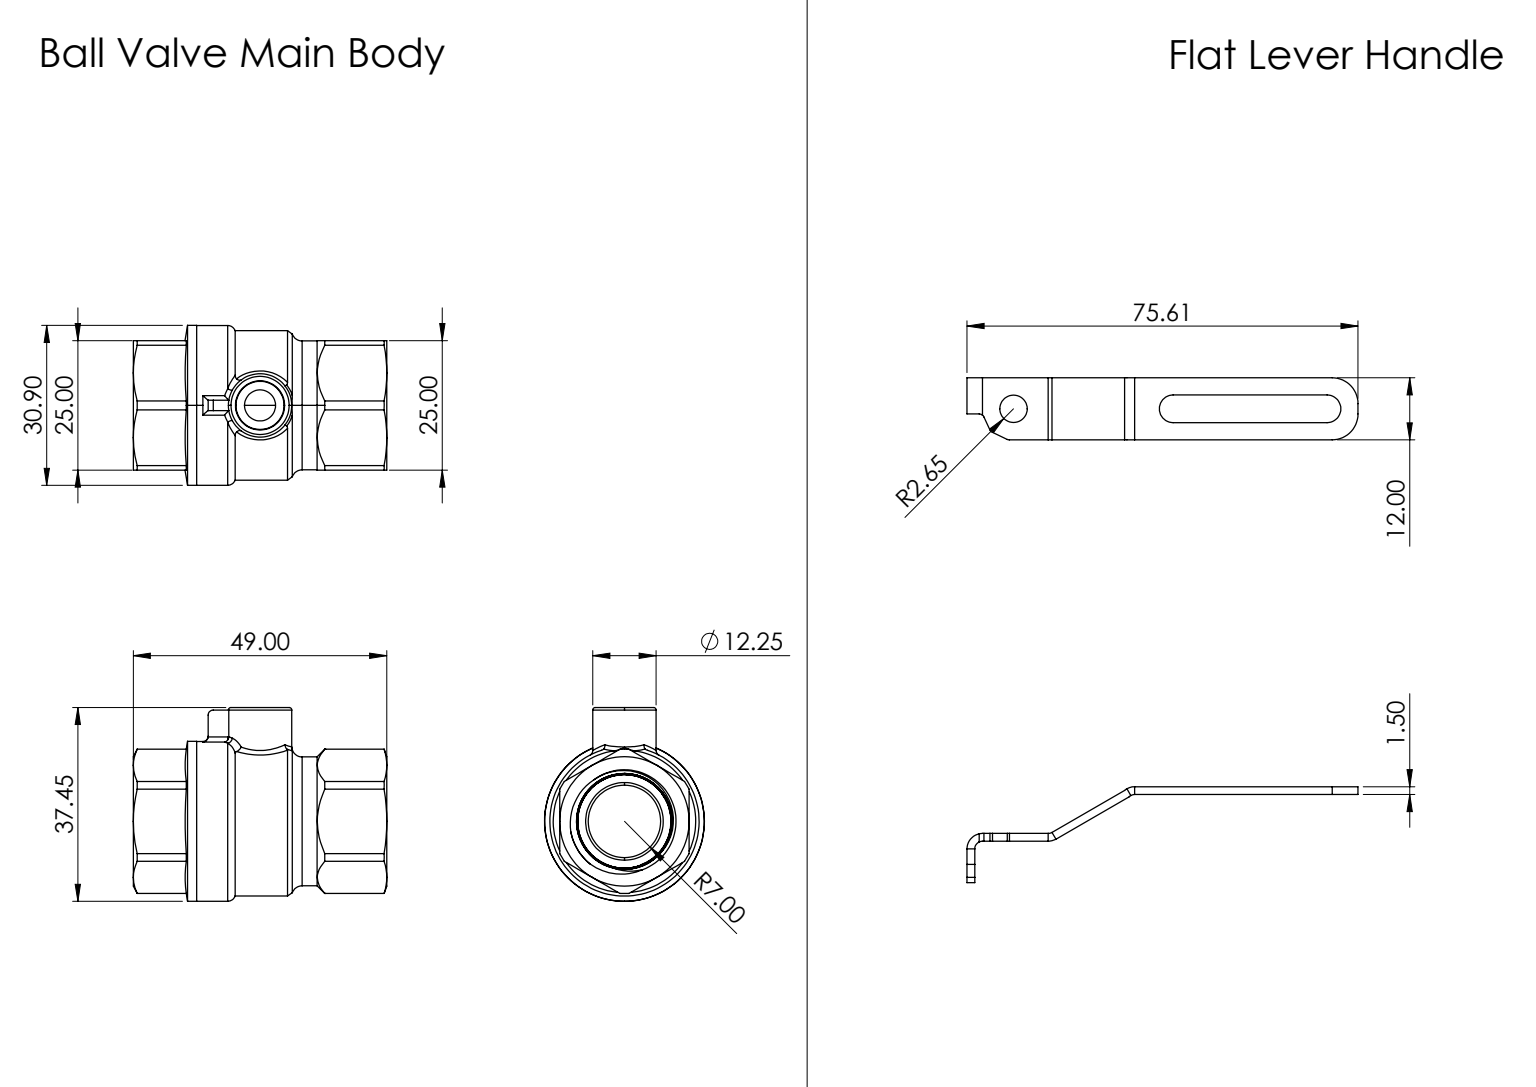
ISO-10303-21;
HEADER;
FILE_DESCRIPTION (('STEP AP214'),
    '1' );
FILE_NAME ('Flat Lever Handle.step',
    '2026-10-09T13:48:35',
    ( '' ),
    ( '' ),
    'SwSTEP 2.0',
    'SolidWorks 2026',
    '' );
FILE_SCHEMA (( 'AUTOMOTIVE_DESIGN' ));
ENDSEC;

DATA;
#4=DIRECTION ( 'NONE',  ( 1.000000000000000000, 0.000000000000000000, 0.000000000000000000 ) ) ;
#6=EDGE_LOOP ( 'NONE', ( #5081, #3644, #13220, #12725 ) ) ;
#25=AXIS2_PLACEMENT_3D ( 'NONE', #17058, #6275, #4594 ) ;
#141=CARTESIAN_POINT ( 'NONE',  ( -130.2348000000000070, 19.50000000000000000, -2.000000000000000000 ) ) ;
#152=CIRCLE ( 'NONE', #7126, 1.500000000000001332 ) ;
#154=EDGE_CURVE ( 'NONE', #7280, #18990, #3410, .T. ) ;
#165=VERTEX_POINT ( 'NONE', #14005 ) ;
#197=DIRECTION ( 'NONE',  ( 0.000000000000000000, 1.000000000000000000, 0.000000000000000000 ) ) ;
#205=ORIENTED_EDGE ( 'NONE', *, *, #8949, .F. ) ;
#208=EDGE_CURVE ( 'NONE', #14474, #22330, #6328, .T. ) ;
#229=DIRECTION ( 'NONE',  ( -0.5000000000000169864, 0.8660254037844288266, 0.000000000000000000 ) ) ;
#230=ORIENTED_EDGE ( 'NONE', *, *, #502, .T. ) ;
#262=LINE ( 'NONE', #11311, #3334 ) ;
#289=DIRECTION ( 'NONE',  ( 1.000000000000000000, 0.000000000000000000, 0.000000000000000000 ) ) ;
#311=VECTOR ( 'NONE', #7009, 1000.000000000000000 ) ;
#329=FACE_OUTER_BOUND ( 'NONE', #10599, .T. ) ;
#332=CYLINDRICAL_SURFACE ( 'NONE', #6125, 2.649999999999999911 ) ;
#336=CLOSED_SHELL ( 'NONE', ( #19786, #22741, #8979, #14137, #5705, #10585, #19906, #17710, #15034, #14866, #16344, #2572, #1995, #20352, #20018, #16952, #22187, #19348, #3814, #13211, #2540, #15971, #923, #17120, #9106, #4929, #6763, #19413, #8384, #21247, #11430, #1672, #12020, #13623, #15533, #9283, #9847, #3649, #4205, #7320, #9527, #23189, #20165, #21835, #18823, #16204, #1398 ) ) ;
#371=PLANE ( 'NONE',  #4207 ) ;
#399=ORIENTED_EDGE ( 'NONE', *, *, #17076, .T. ) ;
#408=CARTESIAN_POINT ( 'NONE',  ( -9.000000000000000000, 19.50000000000000000, -1.000000000000000000 ) ) ;
#412=AXIS2_PLACEMENT_3D ( 'NONE', #8961, #23955, #5663 ) ;
#424=CARTESIAN_POINT ( 'NONE',  ( 23.75352077758000036, 36.75000000000000000, 6.000000000000000000 ) ) ;
#427=CYLINDRICAL_SURFACE ( 'NONE', #12766, 2.999999999999999112 ) ;
#434=FACE_OUTER_BOUND ( 'NONE', #19147, .T. ) ;
#470=DIRECTION ( 'NONE',  ( 0.000000000000000000, 1.000000000000000000, 0.000000000000000000 ) ) ;
#483=PRODUCT ( 'Flat Lever Handle', 'Flat Lever Handle', '', ( #22105 ) ) ;
#502=EDGE_CURVE ( 'NONE', #22896, #18160, #1313, .T. ) ;
#506=CARTESIAN_POINT ( 'NONE',  ( -7.500000000000000000, 22.00000000000000000, 1.000000000000000000 ) ) ;
#512=ORIENTED_EDGE ( 'NONE', *, *, #10459, .F. ) ;
#531=DIRECTION ( 'NONE',  ( 0.8660254037844288266, 0.5000000000000169864, 0.000000000000000000 ) ) ;
#535=CARTESIAN_POINT ( 'NONE',  ( -9.000000000000000000, 18.50000000000000000, -5.000000000000000000 ) ) ;
#537=EDGE_CURVE ( 'NONE', #23889, #15891, #18705, .T. ) ;
#545=ORIENTED_EDGE ( 'NONE', *, *, #18849, .F. ) ;
#560=DIRECTION ( 'NONE',  ( 0.000000000000000000, 0.000000000000000000, -1.000000000000000000 ) ) ;
#582=ORIENTED_EDGE ( 'NONE', *, *, #5142, .F. ) ;
#583=EDGE_CURVE ( 'NONE', #14220, #9013, #21124, .T. ) ;
#589=DIRECTION ( 'NONE',  ( -0.5000000000000169864, 0.8660254037844288266, 0.000000000000000000 ) ) ;
#611=VERTEX_POINT ( 'NONE', #13485 ) ;
#615=ORIENTED_EDGE ( 'NONE', *, *, #5201, .F. ) ;
#634=EDGE_CURVE ( 'NONE', #15280, #17036, #9741, .T. ) ;
#637=CARTESIAN_POINT ( 'NONE',  ( 23.41677564524290744, 35.51856778792605240, -6.000000000000000000 ) ) ;
#640=ORIENTED_EDGE ( 'NONE', *, *, #17076, .F. ) ;
#641=CYLINDRICAL_SURFACE ( 'NONE', #10623, 1.000000000000000888 ) ;
#653=CARTESIAN_POINT ( 'NONE',  ( 7.446152422707000618, 28.20096189432300093, 6.000000000000000000 ) ) ;
#677=ORIENTED_EDGE ( 'NONE', *, *, #17568, .T. ) ;
#722=PLANE ( 'NONE',  #6401 ) ;
#728=ORIENTED_EDGE ( 'NONE', *, *, #1649, .T. ) ;
#729=VECTOR ( 'NONE', #20922, 1000.000000000000000 ) ;
#732=DIRECTION ( 'NONE',  ( 0.000000000000000000, -1.000000000000000000, 1.361873576874000145E-14 ) ) ;
#734=AXIS2_PLACEMENT_3D ( 'NONE', #10520, #4708, #10636 ) ;
#736=DIRECTION ( 'NONE',  ( 0.8660254037844288266, 0.5000000000000169864, 0.000000000000000000 ) ) ;
#773=DIRECTION ( 'NONE',  ( 0.000000000000000000, -1.000000000000000000, 0.000000000000000000 ) ) ;
#789=FACE_OUTER_BOUND ( 'NONE', #3552, .T. ) ;
#793=FACE_OUTER_BOUND ( 'NONE', #14111, .T. ) ;
#808=EDGE_CURVE ( 'NONE', #11090, #23810, #13051, .T. ) ;
#823=ORIENTED_EDGE ( 'NONE', *, *, #5689, .F. ) ;
#860=CARTESIAN_POINT ( 'NONE',  ( -6.000000000000000000, 28.00000000000000000, 1.229194263906999929 ) ) ;
#864=CARTESIAN_POINT ( 'NONE',  ( 7.446152422707000618, 28.20096189432300093, -6.000000000000000000 ) ) ;
#881=LINE ( 'NONE', #11679, #5311 ) ;
#923=ADVANCED_FACE ( 'NONE', ( #1624 ), #23661, .F. ) ;
#932=VECTOR ( 'NONE', #12319, 1000.000000000000000 ) ;
#962=FACE_OUTER_BOUND ( 'NONE', #5721, .T. ) ;
#983=PLANE ( 'NONE',  #23592 ) ;
#1009=CIRCLE ( 'NONE', #16482, 5.000000000000000000 ) ;
#1013=CARTESIAN_POINT ( 'NONE',  ( 23.41677564524290744, 34.01856778792605240, 6.000000000000000000 ) ) ;
#1042=CARTESIAN_POINT ( 'NONE',  ( 60.61494135913342518, 27.01856778792605240, -2.673746900119611247 ) ) ;
#1047=AXIS2_PLACEMENT_3D ( 'NONE', #19546, #12406, #6941 ) ;
#1061=DIRECTION ( 'NONE',  ( 1.000000000000000000, 0.000000000000000000, -1.253337711393242021E-14 ) ) ;
#1093=DIRECTION ( 'NONE',  ( 1.000000000000000000, 0.000000000000000000, 0.000000000000000000 ) ) ;
#1107=VECTOR ( 'NONE', #14524, 1000.000000000000000 ) ;
#1126=ORIENTED_EDGE ( 'NONE', *, *, #3156, .T. ) ;
#1130=ORIENTED_EDGE ( 'NONE', *, *, #7876, .F. ) ;
#1136=CARTESIAN_POINT ( 'NONE',  ( -3.657438266360000245, 28.00000000000000000, 3.657438266360000245 ) ) ;
#1226=CARTESIAN_POINT ( 'NONE',  ( 30.87226923053214378, 37.01856778792605240, -2.673746900119611247 ) ) ;
#1243=CARTESIAN_POINT ( 'NONE',  ( -7.500000000000000000, 18.50000000000000000, -5.000000000000000000 ) ) ;
#1253=ORIENTED_EDGE ( 'NONE', *, *, #13521, .F. ) ;
#1276=EDGE_CURVE ( 'NONE', #9702, #13003, #19100, .T. ) ;
#1285=ORIENTED_EDGE ( 'NONE', *, *, #583, .F. ) ;
#1290=ORIENTED_EDGE ( 'NONE', *, *, #154, .F. ) ;
#1301=DIRECTION ( 'NONE',  ( 0.000000000000000000, 0.000000000000000000, -1.000000000000000000 ) ) ;
#1313=CIRCLE ( 'NONE', #11367, 0.9999999999999995559 ) ;
#1318=FACE_OUTER_BOUND ( 'NONE', #12289, .T. ) ;
#1332=AXIS2_PLACEMENT_3D ( 'NONE', #10810, #12736, #5236 ) ;
#1336=ORIENTED_EDGE ( 'NONE', *, *, #20077, .F. ) ;
#1348=EDGE_LOOP ( 'NONE', ( #23222, #2521, #7520, #9139 ) ) ;
#1352=FACE_OUTER_BOUND ( 'NONE', #11148, .T. ) ;
#1359=DIRECTION ( 'NONE',  ( 0.000000000000000000, 0.000000000000000000, 1.000000000000000000 ) ) ;
#1360=VERTEX_POINT ( 'NONE', #23263 ) ;
#1373=CARTESIAN_POINT ( 'NONE',  ( -9.000000000000000000, 19.50000000000000000, -1.000000000000000000 ) ) ;
#1398=ADVANCED_FACE ( 'NONE', ( #18306 ), #5347, .F. ) ;
#1449=ORIENTED_EDGE ( 'NONE', *, *, #13356, .F. ) ;
#1459=CARTESIAN_POINT ( 'NONE',  ( 23.41677564524290744, 37.01856778792605240, -6.000000000000000000 ) ) ;
#1470=ORIENTED_EDGE ( 'NONE', *, *, #634, .T. ) ;
#1529=AXIS2_PLACEMENT_3D ( 'NONE', #6973, #16287, #9266 ) ;
#1538=FACE_OUTER_BOUND ( 'NONE', #11239, .T. ) ;
#1541=EDGE_CURVE ( 'NONE', #13175, #5360, #5876, .T. ) ;
#1546=CARTESIAN_POINT ( 'NONE',  ( 2.649999999999999911, 28.00000000000000000, 0.000000000000000000 ) ) ;
#1571=CYLINDRICAL_SURFACE ( 'NONE', #15011, 2.673746900119611247 ) ;
#1576=CARTESIAN_POINT ( 'NONE',  ( 66.60588651278291650, 37.01856778792605240, 1.000000000000000000 ) ) ;
#1602=CARTESIAN_POINT ( 'NONE',  ( 60.61494135913342518, 27.01856778792605240, 2.673746900119611247 ) ) ;
#1616=ORIENTED_EDGE ( 'NONE', *, *, #7937, .F. ) ;
#1619=DIRECTION ( 'NONE',  ( 0.000000000000000000, 1.000000000000000000, 0.000000000000000000 ) ) ;
#1621=ORIENTED_EDGE ( 'NONE', *, *, #21569, .T. ) ;
#1624=FACE_OUTER_BOUND ( 'NONE', #21156, .T. ) ;
#1625=ORIENTED_EDGE ( 'NONE', *, *, #4322, .T. ) ;
#1639=ORIENTED_EDGE ( 'NONE', *, *, #2556, .F. ) ;
#1649=EDGE_CURVE ( 'NONE', #13003, #12335, #9333, .T. ) ;
#1667=EDGE_LOOP ( 'NONE', ( #1625, #4186, #23393, #4526 ) ) ;
#1671=EDGE_LOOP ( 'NONE', ( #5379, #9334, #2085, #16002 ) ) ;
#1672=ADVANCED_FACE ( 'NONE', ( #11276 ), #14887, .F. ) ;
#1674=CARTESIAN_POINT ( 'NONE',  ( -6.637070260807000466, 27.93157662065900126, 1.000000000000000000 ) ) ;
#1689=FACE_BOUND ( 'NONE', #22379, .T. ) ;
#1737=EDGE_CURVE ( 'NONE', #1360, #17036, #8351, .T. ) ;
#1739=CIRCLE ( 'NONE', #12188, 1.000000000000000888 ) ;
#1756=ORIENTED_EDGE ( 'NONE', *, *, #16140, .T. ) ;
#1764=VECTOR ( 'NONE', #4364, 1000.000000000000000 ) ;
#1771=EDGE_CURVE ( 'NONE', #6372, #15650, #8993, .T. ) ;
#1792=DIRECTION ( 'NONE',  ( 0.000000000000000000, 0.000000000000000000, 1.000000000000000000 ) ) ;
#1824=ORIENTED_EDGE ( 'NONE', *, *, #23121, .T. ) ;
#1840=PLANE ( 'NONE',  #16418 ) ;
#1847=CARTESIAN_POINT ( 'NONE',  ( -7.500000000000000000, 18.50000000000000000, -2.000000000000000000 ) ) ;
#1861=DIRECTION ( 'NONE',  ( 0.000000000000000000, -1.000000000000000000, 0.000000000000000000 ) ) ;
#1876=MECHANICAL_DESIGN_GEOMETRIC_PRESENTATION_REPRESENTATION('',(#8060),#12344);
#1896=DIRECTION ( 'NONE',  ( -0.000000000000000000, 1.000000000000000000, -0.000000000000000000 ) ) ;
#1905=VECTOR ( 'NONE', #20072, 1000.000000000000000 ) ;
#1971=ORIENTED_EDGE ( 'NONE', *, *, #154, .T. ) ;
#1977=EDGE_CURVE ( 'NONE', #5360, #13125, #15211, .T. ) ;
#1995=ADVANCED_FACE ( 'NONE', ( #2386 ), #3858, .F. ) ;
#1998=PRODUCT_DEFINITION_CONTEXT ( 'detailed design', #23802, 'design' ) ;
#2000=DIRECTION ( 'NONE',  ( 0.000000000000000000, -1.000000000000000000, 0.000000000000000000 ) ) ;
#2012=LINE ( 'NONE', #23616, #6899 ) ;
#2020=CARTESIAN_POINT ( 'NONE',  ( -3.657438266360000245, 26.50000000000000000, 3.657438266360000245 ) ) ;
#2038=DIRECTION ( 'NONE',  ( 0.000000000000000000, -1.000000000000000000, 0.000000000000000000 ) ) ;
#2085=ORIENTED_EDGE ( 'NONE', *, *, #10886, .T. ) ;
#2090=ORIENTED_EDGE ( 'NONE', *, *, #3850, .F. ) ;
#2136=CARTESIAN_POINT ( 'NONE',  ( -6.525832981339341643, 26.41017609473133732, 0.9999999999999872324 ) ) ;
#2157=PLANE ( 'NONE',  #9897 ) ;
#2190=CARTESIAN_POINT ( 'NONE',  ( 60.61494135913342518, 35.51856778792605240, 2.673746900119610359 ) ) ;
#2196=DIRECTION ( 'NONE',  ( 0.000000000000000000, 0.000000000000000000, -1.000000000000000000 ) ) ;
#2205=DIRECTION ( 'NONE',  ( 0.000000000000000000, -1.000000000000000000, 0.000000000000000000 ) ) ;
#2209=DIRECTION ( 'NONE',  ( 0.000000000000000000, 0.000000000000000000, 1.000000000000000000 ) ) ;
#2241=DIRECTION ( 'NONE',  ( 1.000000000000000000, 0.000000000000000000, 0.000000000000000000 ) ) ;
#2243=ORIENTED_EDGE ( 'NONE', *, *, #13378, .T. ) ;
#2262=CIRCLE ( 'NONE', #11164, 1.500000000000001332 ) ;
#2276=VECTOR ( 'NONE', #589, 1000.000000000000114 ) ;
#2284=ORIENTED_EDGE ( 'NONE', *, *, #20180, .T. ) ;
#2317=CARTESIAN_POINT ( 'NONE',  ( 23.01485185659291233, 37.01856778792605240, -6.000000000000000000 ) ) ;
#2318=ORIENTED_EDGE ( 'NONE', *, *, #537, .T. ) ;
#2350=DIRECTION ( 'NONE',  ( 0.000000000000000000, -1.000000000000000000, 0.000000000000000000 ) ) ;
#2356=DIRECTION ( 'NONE',  ( -1.387778780781444413E-14, 1.000000000000000000, 0.000000000000000000 ) ) ;
#2373=DIRECTION ( 'NONE',  ( 0.000000000000000000, 0.000000000000000000, -1.000000000000000000 ) ) ;
#2374=VERTEX_POINT ( 'NONE', #18954 ) ;
#2386=FACE_OUTER_BOUND ( 'NONE', #10840, .T. ) ;
#2399=CARTESIAN_POINT ( 'NONE',  ( -6.637070260807000466, 26.35799170939839797, 1.000000000000000000 ) ) ;
#2425=DIRECTION ( 'NONE',  ( 0.9063077870366409439, 0.000000000000000000, -0.4226182617407189257 ) ) ;
#2465=CARTESIAN_POINT ( 'NONE',  ( 8.196152422706999729, 26.90192378864669820, -6.000000000000000000 ) ) ;
#2473=AXIS2_PLACEMENT_3D ( 'NONE', #2819, #1359, #21464 ) ;
#2501=AXIS2_PLACEMENT_3D ( 'NONE', #7515, #2425, #9577 ) ;
#2521=ORIENTED_EDGE ( 'NONE', *, *, #18719, .F. ) ;
#2529=VECTOR ( 'NONE', #15495, 1000.000000000000000 ) ;
#2540=ADVANCED_FACE ( 'NONE', ( #23055 ), #15665, .T. ) ;
#2556=EDGE_CURVE ( 'NONE', #18990, #5263, #11534, .T. ) ;
#2572=ADVANCED_FACE ( 'NONE', ( #3789 ), #13104, .F. ) ;
#2591=CARTESIAN_POINT ( 'NONE',  ( -7.500000000000000000, 22.00000000000000000, 1.000000000000000000 ) ) ;
#2603=AXIS2_PLACEMENT_3D ( 'NONE', #5656, #9656, #20438 ) ;
#2616=LINE ( 'NONE', #8311, #4226 ) ;
#2620=CARTESIAN_POINT ( 'NONE',  ( -6.199443458293737663, 26.48693030808626503, 1.100246419409809828 ) ) ;
#2655=PLANE ( 'NONE',  #4969 ) ;
#2658=DIRECTION ( 'NONE',  ( 0.000000000000000000, 1.000000000000000000, 0.000000000000000000 ) ) ;
#2660=ORIENTED_EDGE ( 'NONE', *, *, #12790, .F. ) ;
#2681=VERTEX_POINT ( 'NONE', #13452 ) ;
#2688=CARTESIAN_POINT ( 'NONE',  ( 7.446152422707000618, 28.20096189432300093, -6.000000000000000000 ) ) ;
#2740=EDGE_CURVE ( 'NONE', #23570, #10530, #10318, .T. ) ;
#2786=CIRCLE ( 'NONE', #16311, 1.000000000000000222 ) ;
#2800=CARTESIAN_POINT ( 'NONE',  ( -8.250000000000000000, 18.50000000000000000, 0.000000000000000000 ) ) ;
#2801=AXIS2_PLACEMENT_3D ( 'NONE', #22276, #7504, #4242 ) ;
#2809=CARTESIAN_POINT ( 'NONE',  ( 66.60588651278291650, 37.01856778792605240, -1.000000000000000000 ) ) ;
#2819=CARTESIAN_POINT ( 'NONE',  ( 6.696152422707000618, 29.50000000000000000, 6.000000000000000000 ) ) ;
#2875=VERTEX_POINT ( 'NONE', #21586 ) ;
#2899=PLANE ( 'NONE',  #5691 ) ;
#2914=ORIENTED_EDGE ( 'NONE', *, *, #10159, .F. ) ;
#2929=DIRECTION ( 'NONE',  ( -1.000000000000000000, 0.000000000000000000, 0.000000000000000000 ) ) ;
#2943=CARTESIAN_POINT ( 'NONE',  ( 30.87226923053214378, 27.01856778792605240, -2.673746900119611247 ) ) ;
#2958=CARTESIAN_POINT ( 'NONE',  ( 6.696152422707000618, 26.50000000000000000, 6.000000000000000000 ) ) ;
#2963=CIRCLE ( 'NONE', #7200, 1.000000000000000666 ) ;
#2968=PLANE ( 'NONE',  #7688 ) ;
#2994=LINE ( 'NONE', #17643, #6347 ) ;
#3126=DIRECTION ( 'NONE',  ( 0.000000000000000000, 1.000000000000000000, 0.000000000000000000 ) ) ;
#3138=ORIENTED_EDGE ( 'NONE', *, *, #19897, .F. ) ;
#3145=VECTOR ( 'NONE', #15592, 1000.000000000000114 ) ;
#3156=EDGE_CURVE ( 'NONE', #13296, #15891, #23861, .T. ) ;
#3168=DIRECTION ( 'NONE',  ( 0.4226182617407188702, 0.000000000000000000, 0.9063077870366409439 ) ) ;
#3175=ORIENTED_EDGE ( 'NONE', *, *, #6427, .T. ) ;
#3190=CARTESIAN_POINT ( 'NONE',  ( -0.7783053373570000266, 28.00000000000000000, 5.000000000000000000 ) ) ;
#3204=CARTESIAN_POINT ( 'NONE',  ( 61.60588651278290939, 35.51856778792605240, -1.000000000000000000 ) ) ;
#3234=CARTESIAN_POINT ( 'NONE',  ( 6.696152422707000618, 29.50000000000000000, 115.0195023120000002 ) ) ;
#3270=DIRECTION ( 'NONE',  ( 0.000000000000000000, 0.000000000000000000, 1.000000000000000000 ) ) ;
#3290=CARTESIAN_POINT ( 'NONE',  ( 61.60588651278290939, 35.51856778792605240, -6.000000000000000000 ) ) ;
#3316=VERTEX_POINT ( 'NONE', #10412 ) ;
#3334=VECTOR ( 'NONE', #22437, 1000.000000000000000 ) ;
#3337=SURFACE_STYLE_FILL_AREA ( #19920 ) ;
#3359=ORIENTED_EDGE ( 'NONE', *, *, #3772, .T. ) ;
#3407=LINE ( 'NONE', #3520, #1107 ) ;
#3410=CIRCLE ( 'NONE', #16911, 2.673746900119611247 ) ;
#3432=DIRECTION ( 'NONE',  ( 0.000000000000000000, 1.000000000000000000, 0.000000000000000000 ) ) ;
#3455=( NAMED_UNIT ( * ) SI_UNIT ( $, .STERADIAN. ) SOLID_ANGLE_UNIT ( ) );
#3457=DIRECTION ( 'NONE',  ( 0.000000000000000000, 0.000000000000000000, -1.000000000000000000 ) ) ;
#3459=CIRCLE ( 'NONE', #22010, 3.000000000000002665 ) ;
#3477=VECTOR ( 'NONE', #17700, 1000.000000000000000 ) ;
#3499=VECTOR ( 'NONE', #9426, 1000.000000000000000 ) ;
#3512=DIRECTION ( 'NONE',  ( 0.000000000000000000, 0.000000000000000000, -1.000000000000000000 ) ) ;
#3520=CARTESIAN_POINT ( 'NONE',  ( -4.563746053395999702, 28.00000000000000000, 4.080056528100000079 ) ) ;
#3552=EDGE_LOOP ( 'NONE', ( #5007, #17455, #1130, #8586, #15007, #13159 ) ) ;
#3555=LINE ( 'NONE', #16264, #18147 ) ;
#3578=ORIENTED_EDGE ( 'NONE', *, *, #5131, .T. ) ;
#3585=ORIENTED_EDGE ( 'NONE', *, *, #23747, .F. ) ;
#3587=CARTESIAN_POINT ( 'NONE',  ( 61.60588651278290939, 37.01856778792605240, -6.000000000000000000 ) ) ;
#3593=EDGE_CURVE ( 'NONE', #17322, #5263, #2994, .T. ) ;
#3608=EDGE_CURVE ( 'NONE', #15241, #18990, #17892, .T. ) ;
#3625=FACE_OUTER_BOUND ( 'NONE', #1667, .T. ) ;
#3633=VERTEX_POINT ( 'NONE', #6978 ) ;
#3644=ORIENTED_EDGE ( 'NONE', *, *, #8463, .T. ) ;
#3649=ADVANCED_FACE ( 'NONE', ( #1538 ), #19826, .F. ) ;
#3696=DIRECTION ( 'NONE',  ( 0.000000000000000000, 0.000000000000000000, 1.000000000000000000 ) ) ;
#3707=PLANE ( 'NONE',  #14292 ) ;
#3708=EDGE_CURVE ( 'NONE', #3316, #12335, #152, .T. ) ;
#3758=DIRECTION ( 'NONE',  ( 1.000000000000000000, 0.000000000000000000, 0.000000000000000000 ) ) ;
#3772=EDGE_CURVE ( 'NONE', #7943, #18240, #18595, .T. ) ;
#3784=DIRECTION ( 'NONE',  ( 0.000000000000000000, 0.000000000000000000, 1.000000000000000000 ) ) ;
#3789=FACE_OUTER_BOUND ( 'NONE', #18293, .T. ) ;
#3793=CYLINDRICAL_SURFACE ( 'NONE', #23685, 1.000000000000000000 ) ;
#3814=ADVANCED_FACE ( 'NONE', ( #22572 ), #641, .T. ) ;
#3829=LINE ( 'NONE', #13469, #6944 ) ;
#3836=CARTESIAN_POINT ( 'NONE',  ( 6.696152422707000618, 29.50000000000000000, 115.0195023120000002 ) ) ;
#3841=DIRECTION ( 'NONE',  ( 0.000000000000000000, -1.000000000000000000, 0.000000000000000000 ) ) ;
#3850=EDGE_CURVE ( 'NONE', #5360, #14220, #13360, .T. ) ;
#3854=VECTOR ( 'NONE', #3784, 1000.000000000000000 ) ;
#3858=PLANE ( 'NONE',  #21283 ) ;
#3860=ORIENTED_EDGE ( 'NONE', *, *, #13378, .F. ) ;
#3861=DIRECTION ( 'NONE',  ( 0.000000000000000000, 0.000000000000000000, 1.000000000000000000 ) ) ;
#3875=CARTESIAN_POINT ( 'NONE',  ( -7.500000000000000000, 24.99999999999999645, 1.000000000000000000 ) ) ;
#3891=DIRECTION ( 'NONE',  ( 0.000000000000000000, -1.000000000000000000, 0.000000000000000000 ) ) ;
#3910=ORIENTED_EDGE ( 'NONE', *, *, #4655, .T. ) ;
#3937=ORIENTED_EDGE ( 'NONE', *, *, #5491, .T. ) ;
#3968=ORIENTED_EDGE ( 'NONE', *, *, #10594, .T. ) ;
#3976=FACE_OUTER_BOUND ( 'NONE', #19466, .T. ) ;
#3996=CARTESIAN_POINT ( 'NONE',  ( 61.60588651278290939, 74.97299614839606363, 1.000000000000000000 ) ) ;
#4018=ORIENTED_EDGE ( 'NONE', *, *, #2556, .T. ) ;
#4132=FACE_OUTER_BOUND ( 'NONE', #23776, .T. ) ;
#4159=VECTOR ( 'NONE', #21288, 1000.000000000000000 ) ;
#4186=ORIENTED_EDGE ( 'NONE', *, *, #12227, .F. ) ;
#4205=ADVANCED_FACE ( 'NONE', ( #434 ), #12923, .F. ) ;
#4207=AXIS2_PLACEMENT_3D ( 'NONE', #2317, #18674, #13574 ) ;
#4226=VECTOR ( 'NONE', #21278, 1000.000000000000000 ) ;
#4242=DIRECTION ( 'NONE',  ( 0.000000000000000000, 0.000000000000000000, -1.000000000000000000 ) ) ;
#4256=CARTESIAN_POINT ( 'NONE',  ( -9.000000000000000000, 22.00000000000000000, 1.000000000000000000 ) ) ;
#4258=CARTESIAN_POINT ( 'NONE',  ( 30.87226923053214378, 37.01856778792605240, 0.000000000000000000 ) ) ;
#4322=EDGE_CURVE ( 'NONE', #6372, #11438, #22241, .T. ) ;
#4332=VECTOR ( 'NONE', #13729, 1000.000000000000000 ) ;
#4341=ORIENTED_EDGE ( 'NONE', *, *, #5144, .T. ) ;
#4364=DIRECTION ( 'NONE',  ( 0.000000000000000000, 0.000000000000000000, 1.000000000000000000 ) ) ;
#4365=CYLINDRICAL_SURFACE ( 'NONE', #15806, 5.000000000000000000 ) ;
#4381=CARTESIAN_POINT ( 'NONE',  ( -1.200923599098000061, 26.50000000000000000, 5.906307787036999990 ) ) ;
#4388=ORIENTED_EDGE ( 'NONE', *, *, #808, .T. ) ;
#4390=AXIS2_PLACEMENT_3D ( 'NONE', #8983, #23856, #3758 ) ;
#4411=CARTESIAN_POINT ( 'NONE',  ( -6.637070260807000466, 28.00000000000000000, 2.000000000000000000 ) ) ;
#4416=CARTESIAN_POINT ( 'NONE',  ( -9.000000000000000000, 24.99999999999999645, 1.000000000000000000 ) ) ;
#4417=VECTOR ( 'NONE', #21401, 1000.000000000000000 ) ;
#4438=CARTESIAN_POINT ( 'NONE',  ( -9.000000000000000000, 18.50000000000000000, -2.000000000000000000 ) ) ;
#4456=ORIENTED_EDGE ( 'NONE', *, *, #22088, .T. ) ;
#4462=EDGE_CURVE ( 'NONE', #2681, #19197, #19467, .T. ) ;
#4472=VECTOR ( 'NONE', #3168, 1000.000000000000000 ) ;
#4488=DIRECTION ( 'NONE',  ( 0.000000000000000000, 0.000000000000000000, -1.000000000000000000 ) ) ;
#4501=LINE ( 'NONE', #15623, #14422 ) ;
#4514=VECTOR ( 'NONE', #531, 1000.000000000000114 ) ;
#4526=ORIENTED_EDGE ( 'NONE', *, *, #16296, .F. ) ;
#4532=ORIENTED_EDGE ( 'NONE', *, *, #20755, .T. ) ;
#4589=PLANE ( 'NONE',  #13873 ) ;
#4594=DIRECTION ( 'NONE',  ( 0.5000000000000172085, -0.8660254037844288266, 0.000000000000000000 ) ) ;
#4598=DIRECTION ( 'NONE',  ( 0.000000000000000000, -1.000000000000000000, 0.000000000000000000 ) ) ;
#4602=CARTESIAN_POINT ( 'NONE',  ( 6.696152422707000618, 26.50000000000000000, -6.000000000000000000 ) ) ;
#4639=DIRECTION ( 'NONE',  ( -1.000000000000000000, 0.000000000000000000, 0.000000000000000000 ) ) ;
#4644=LINE ( 'NONE', #6203, #14553 ) ;
#4650=ORIENTED_EDGE ( 'NONE', *, *, #20761, .T. ) ;
#4655=EDGE_CURVE ( 'NONE', #18177, #23789, #8686, .T. ) ;
#4666=VERTEX_POINT ( 'NONE', #6737 ) ;
#4668=FACE_OUTER_BOUND ( 'NONE', #6237, .T. ) ;
#4676=CARTESIAN_POINT ( 'NONE',  ( -8.250000000000000000, 23.50000000000000000, 1.000000000000000000 ) ) ;
#4688=EDGE_CURVE ( 'NONE', #13175, #16279, #18015, .T. ) ;
#4693=DIRECTION ( 'NONE',  ( -0.000000000000000000, 1.000000000000000000, -0.000000000000000000 ) ) ;
#4696=DIRECTION ( 'NONE',  ( -1.000000000000000000, 0.000000000000000000, 0.000000000000000000 ) ) ;
#4708=DIRECTION ( 'NONE',  ( 1.000000000000000000, 0.000000000000000000, 0.000000000000000000 ) ) ;
#4716=ORIENTED_EDGE ( 'NONE', *, *, #7876, .T. ) ;
#4733=ORIENTED_EDGE ( 'NONE', *, *, #9700, .F. ) ;
#4748=DIRECTION ( 'NONE',  ( 0.000000000000000000, 1.000000000000000000, 0.000000000000000000 ) ) ;
#4758=ORIENTED_EDGE ( 'NONE', *, *, #21648, .F. ) ;
#4774=EDGE_LOOP ( 'NONE', ( #11243, #10368, #13428, #5434, #582, #17464 ) ) ;
#4814=EDGE_LOOP ( 'NONE', ( #22596, #17054, #2284, #8840 ) ) ;
#4876=DIRECTION ( 'NONE',  ( 1.000000000000000000, 0.000000000000000000, 0.000000000000000000 ) ) ;
#4901=ORIENTED_EDGE ( 'NONE', *, *, #18157, .F. ) ;
#4929=ADVANCED_FACE ( 'NONE', ( #22576 ), #11570, .T. ) ;
#4955=EDGE_CURVE ( 'NONE', #13125, #9013, #13607, .T. ) ;
#4969=AXIS2_PLACEMENT_3D ( 'NONE', #21430, #15838, #4598 ) ;
#4985=CIRCLE ( 'NONE', #13863, 1.000000000000000000 ) ;
#4991=VECTOR ( 'NONE', #7255, 1000.000000000000000 ) ;
#5007=ORIENTED_EDGE ( 'NONE', *, *, #9700, .T. ) ;
#5037=SURFACE_SIDE_STYLE ('',( #3337 ) ) ;
#5053=VERTEX_POINT ( 'NONE', #15902 ) ;
#5081=ORIENTED_EDGE ( 'NONE', *, *, #11891, .T. ) ;
#5108=CARTESIAN_POINT ( 'NONE',  ( -4.080056528100000079, 26.50000000000000000, 4.563746053395999702 ) ) ;
#5110=ORIENTED_EDGE ( 'NONE', *, *, #13519, .F. ) ;
#5117=CARTESIAN_POINT ( 'NONE',  ( 8.196152422706999729, 26.90192378864669820, -6.000000000000000000 ) ) ;
#5119=CARTESIAN_POINT ( 'NONE',  ( -7.625774495095999583, 27.25000000000000000, 1.000000000000000000 ) ) ;
#5131=EDGE_CURVE ( 'NONE', #12555, #13009, #6306, .T. ) ;
#5142=EDGE_CURVE ( 'NONE', #5053, #2374, #2786, .T. ) ;
#5144=EDGE_CURVE ( 'NONE', #21343, #1360, #13449, .T. ) ;
#5166=FACE_OUTER_BOUND ( 'NONE', #21138, .T. ) ;
#5185=FACE_OUTER_BOUND ( 'NONE', #9004, .T. ) ;
#5201=EDGE_CURVE ( 'NONE', #4666, #15717, #9742, .T. ) ;
#5214=CARTESIAN_POINT ( 'NONE',  ( -7.500000000000000000, 19.50000000000000000, -1.000000000000000000 ) ) ;
#5234=AXIS2_PLACEMENT_3D ( 'NONE', #23834, #5554, #5444 ) ;
#5236=DIRECTION ( 'NONE',  ( 1.000000000000000000, 0.000000000000000000, 0.000000000000000000 ) ) ;
#5257=EDGE_CURVE ( 'NONE', #10530, #11734, #10916, .T. ) ;
#5263=VERTEX_POINT ( 'NONE', #1226 ) ;
#5279=AXIS2_PLACEMENT_3D ( 'NONE', #3234, #10617, #9028 ) ;
#5287=ORIENTED_EDGE ( 'NONE', *, *, #7317, .T. ) ;
#5306=CARTESIAN_POINT ( 'NONE',  ( 61.60588651278290939, 37.01856778792605240, 6.000000000000000000 ) ) ;
#5311=VECTOR ( 'NONE', #9857, 1000.000000000000000 ) ;
#5313=ORIENTED_EDGE ( 'NONE', *, *, #8949, .T. ) ;
#5319=FACE_OUTER_BOUND ( 'NONE', #9179, .T. ) ;
#5321=DIRECTION ( 'NONE',  ( 0.000000000000000000, -1.000000000000000000, -1.361873576874000145E-14 ) ) ;
#5325=PLANE ( 'NONE',  #5234 ) ;
#5343=ORIENTED_EDGE ( 'NONE', *, *, #20761, .F. ) ;
#5347=PLANE ( 'NONE',  #1332 ) ;
#5360=VERTEX_POINT ( 'NONE', #3875 ) ;
#5379=ORIENTED_EDGE ( 'NONE', *, *, #17073, .F. ) ;
#5389=EDGE_CURVE ( 'NONE', #13003, #9532, #15477, .T. ) ;
#5396=ORIENTED_EDGE ( 'NONE', *, *, #208, .T. ) ;
#5434=ORIENTED_EDGE ( 'NONE', *, *, #10594, .F. ) ;
#5441=FACE_OUTER_BOUND ( 'NONE', #11137, .T. ) ;
#5444=DIRECTION ( 'NONE',  ( 0.000000000000000000, -1.000000000000000000, 0.000000000000000000 ) ) ;
#5491=EDGE_CURVE ( 'NONE', #23570, #17036, #21318, .T. ) ;
#5514=DIRECTION ( 'NONE',  ( 1.000000000000000000, 0.000000000000000000, 0.000000000000000000 ) ) ;
#5529=ORIENTED_EDGE ( 'NONE', *, *, #3850, .T. ) ;
#5536=ORIENTED_EDGE ( 'NONE', *, *, #1771, .F. ) ;
#5554=DIRECTION ( 'NONE',  ( 0.000000000000000000, 0.000000000000000000, -1.000000000000000000 ) ) ;
#5557=CARTESIAN_POINT ( 'NONE',  ( -9.000000000000000000, 19.50000000000000000, -6.000000000000000000 ) ) ;
#5576=ORIENTED_EDGE ( 'NONE', *, *, #6427, .F. ) ;
#5605=LINE ( 'NONE', #20617, #14024 ) ;
#5638=DIRECTION ( 'NONE',  ( 0.000000000000000000, 0.000000000000000000, -1.000000000000000000 ) ) ;
#5648=DIRECTION ( 'NONE',  ( -0.4226182617407191477, 0.000000000000000000, 0.9063077870366409439 ) ) ;
#5656=CARTESIAN_POINT ( 'NONE',  ( 23.41677564524290744, 34.01856778792605240, -115.0195023120000002 ) ) ;
#5658=VECTOR ( 'NONE', #20898, 1000.000000000000000 ) ;
#5663=DIRECTION ( 'NONE',  ( 0.000000000000000000, 1.000000000000000000, 0.000000000000000000 ) ) ;
#5689=EDGE_CURVE ( 'NONE', #14083, #2875, #20325, .T. ) ;
#5691=AXIS2_PLACEMENT_3D ( 'NONE', #10046, #10410, #17431 ) ;
#5705=ADVANCED_FACE ( 'NONE', ( #5441 ), #9187, .F. ) ;
#5717=DIRECTION ( 'NONE',  ( 1.000000000000000000, 0.000000000000000000, 0.000000000000000000 ) ) ;
#5721=EDGE_LOOP ( 'NONE', ( #12838, #7284, #1616, #18568 ) ) ;
#5741=AXIS2_PLACEMENT_3D ( 'NONE', #11569, #6097, #9744 ) ;
#5757=PRODUCT_DEFINITION ( 'UNKNOWN', '', #16751, #1998 ) ;
#5767=CYLINDRICAL_SURFACE ( 'NONE', #6154, 1.500000000000000222 ) ;
#5774=CARTESIAN_POINT ( 'NONE',  ( -6.414809095751526691, 26.44559118008276144, 1.018491744841189872 ) ) ;
#5808=DIRECTION ( 'NONE',  ( -0.000000000000000000, -0.000000000000000000, 1.000000000000000000 ) ) ;
#5843=ORIENTED_EDGE ( 'NONE', *, *, #19473, .F. ) ;
#5847=DIRECTION ( 'NONE',  ( 1.000000000000000000, 0.000000000000000000, 0.000000000000000000 ) ) ;
#5864=ORIENTED_EDGE ( 'NONE', *, *, #21648, .T. ) ;
#5866=DIRECTION ( 'NONE',  ( -1.000000000000000000, 0.000000000000000000, 0.000000000000000000 ) ) ;
#5876=CIRCLE ( 'NONE', #15147, 1.500000000000000000 ) ;
#5911=ORIENTED_EDGE ( 'NONE', *, *, #12035, .T. ) ;
#5912=EDGE_CURVE ( 'NONE', #165, #7280, #3829, .T. ) ;
#5944=CARTESIAN_POINT ( 'NONE',  ( 30.87226923053214378, 37.01856778792605240, -2.673746900119611247 ) ) ;
#5977=CARTESIAN_POINT ( 'NONE',  ( -130.2348000000000070, 19.50000000000000000, -5.000000000000000000 ) ) ;
#5984=VECTOR ( 'NONE', #14406, 1000.000000000000000 ) ;
#5985=CARTESIAN_POINT ( 'NONE',  ( 23.41677564524290744, 34.01856778792605240, -6.000000000000000000 ) ) ;
#6003=VERTEX_POINT ( 'NONE', #1243 ) ;
#6017=DIRECTION ( 'NONE',  ( 0.000000000000000000, 0.000000000000000000, -1.000000000000000000 ) ) ;
#6053=ORIENTED_EDGE ( 'NONE', *, *, #8147, .F. ) ;
#6082=VECTOR ( 'NONE', #197, 1000.000000000000000 ) ;
#6084=LINE ( 'NONE', #16998, #20483 ) ;
#6094=DIRECTION ( 'NONE',  ( 1.000000000000000000, 0.000000000000000000, 0.000000000000000000 ) ) ;
#6097=DIRECTION ( 'NONE',  ( 0.000000000000000000, -1.000000000000000000, 0.000000000000000000 ) ) ;
#6105=CARTESIAN_POINT ( 'NONE',  ( -2.649999999999999911, 26.50000000000000000, 0.000000000000000000 ) ) ;
#6115=CARTESIAN_POINT ( 'NONE',  ( 23.41677564524290744, 37.01856778792605240, 6.000000000000000000 ) ) ;
#6121=ORIENTED_EDGE ( 'NONE', *, *, #7630, .T. ) ;
#6125=AXIS2_PLACEMENT_3D ( 'NONE', #9671, #7736, #22497 ) ;
#6153=DIRECTION ( 'NONE',  ( 1.000000000000000000, 0.000000000000000000, 0.000000000000000000 ) ) ;
#6154=AXIS2_PLACEMENT_3D ( 'NONE', #3836, #17142, #19072 ) ;
#6175=CARTESIAN_POINT ( 'NONE',  ( 30.87226923053214378, 35.51856778792605240, -2.673746900119611247 ) ) ;
#6192=LINE ( 'NONE', #13577, #13642 ) ;
#6203=CARTESIAN_POINT ( 'NONE',  ( -9.000000000000000000, 18.50000000000000000, -5.000000000000000000 ) ) ;
#6209=DIRECTION ( 'NONE',  ( -1.000000000000000000, 0.000000000000000000, 0.000000000000000000 ) ) ;
#6214=DIRECTION ( 'NONE',  ( 0.000000000000000000, 0.000000000000000000, 1.000000000000000000 ) ) ;
#6237=EDGE_LOOP ( 'NONE', ( #15655, #9289, #9947, #16870 ) ) ;
#6272=CARTESIAN_POINT ( 'NONE',  ( -6.180252273306864552, 27.99999999999999645, 1.080215919051256579 ) ) ;
#6275=DIRECTION ( 'NONE',  ( 0.000000000000000000, 0.000000000000000000, -1.000000000000000000 ) ) ;
#6306=LINE ( 'NONE', #2809, #12077 ) ;
#6328=CIRCLE ( 'NONE', #17557, 1.000000000000000888 ) ;
#6342=CARTESIAN_POINT ( 'NONE',  ( 23.41677564524290744, 34.01856778792605240, 6.000000000000005329 ) ) ;
#6347=VECTOR ( 'NONE', #4693, 1000.000000000000000 ) ;
#6348=CARTESIAN_POINT ( 'NONE',  ( 22.35132670216752260, 35.07441746931966975, 6.000000000000000000 ) ) ;
#6372=VERTEX_POINT ( 'NONE', #5557 ) ;
#6401=AXIS2_PLACEMENT_3D ( 'NONE', #2800, #10064, #20841 ) ;
#6422=AXIS2_PLACEMENT_3D ( 'NONE', #7169, #6819, #12160 ) ;
#6424=ORIENTED_EDGE ( 'NONE', *, *, #9643, .F. ) ;
#6427=EDGE_CURVE ( 'NONE', #13003, #23889, #17288, .T. ) ;
#6455=ORIENTED_EDGE ( 'NONE', *, *, #1737, .T. ) ;
#6460=EDGE_CURVE ( 'NONE', #5053, #18160, #11725, .T. ) ;
#6492=DIRECTION ( 'NONE',  ( 0.000000000000000000, 0.000000000000000000, 1.000000000000000000 ) ) ;
#6520=ORIENTED_EDGE ( 'NONE', *, *, #6869, .F. ) ;
#6524=CIRCLE ( 'NONE', #15412, 3.000000000000000000 ) ;
#6596=DIRECTION ( 'NONE',  ( 0.000000000000000000, 0.000000000000000000, -1.000000000000000000 ) ) ;
#6631=ORIENTED_EDGE ( 'NONE', *, *, #1771, .T. ) ;
#6692=ORIENTED_EDGE ( 'NONE', *, *, #13837, .T. ) ;
#6694=EDGE_LOOP ( 'NONE', ( #20829, #22838, #1285, #2090 ) ) ;
#6729=ORIENTED_EDGE ( 'NONE', *, *, #2740, .F. ) ;
#6735=CARTESIAN_POINT ( 'NONE',  ( 60.61494135913342518, 37.01856778792605240, 0.000000000000000000 ) ) ;
#6737=CARTESIAN_POINT ( 'NONE',  ( 21.91677564524432853, 36.61664399928019265, 6.000000000000000000 ) ) ;
#6763=ADVANCED_FACE ( 'NONE', ( #16930 ), #332, .F. ) ;
#6770=ORIENTED_EDGE ( 'NONE', *, *, #6838, .T. ) ;
#6775=AXIS2_PLACEMENT_3D ( 'NONE', #9191, #2038, #9428 ) ;
#6776=ORIENTED_EDGE ( 'NONE', *, *, #5912, .F. ) ;
#6782=LINE ( 'NONE', #19759, #4472 ) ;
#6807=AXIS2_PLACEMENT_3D ( 'NONE', #21967, #3457, #1861 ) ;
#6819=DIRECTION ( 'NONE',  ( 0.000000000000000000, 0.000000000000000000, 1.000000000000000000 ) ) ;
#6831=( LENGTH_UNIT ( ) NAMED_UNIT ( * ) SI_UNIT ( .MILLI., .METRE. ) );
#6838=EDGE_CURVE ( 'NONE', #12555, #7943, #19690, .T. ) ;
#6846=ORIENTED_EDGE ( 'NONE', *, *, #7007, .T. ) ;
#6869=EDGE_CURVE ( 'NONE', #23810, #15717, #10400, .T. ) ;
#6898=CARTESIAN_POINT ( 'NONE',  ( -7.500000000000000000, 24.99999999999999645, -6.000000000000000000 ) ) ;
#6899=VECTOR ( 'NONE', #1896, 1000.000000000000000 ) ;
#6906=FACE_OUTER_BOUND ( 'NONE', #7453, .T. ) ;
#6931=VECTOR ( 'NONE', #8000, 1000.000000000000000 ) ;
#6937=ORIENTED_EDGE ( 'NONE', *, *, #21569, .F. ) ;
#6941=DIRECTION ( 'NONE',  ( 1.000000000000000000, 0.000000000000000000, 0.000000000000000000 ) ) ;
#6944=VECTOR ( 'NONE', #20872, 1000.000000000000000 ) ;
#6973=CARTESIAN_POINT ( 'NONE',  ( -6.000000000000000000, 24.99999999999999645, 1.000000000000000000 ) ) ;
#6978=CARTESIAN_POINT ( 'NONE',  ( -2.649999999999999911, 26.50000000000000000, 0.000000000000000000 ) ) ;
#6987=CARTESIAN_POINT ( 'NONE',  ( 22.35132670216743023, 35.07441746931982607, -115.0195023120000002 ) ) ;
#7002=FACE_BOUND ( 'NONE', #14793, .T. ) ;
#7007=EDGE_CURVE ( 'NONE', #18186, #13296, #8465, .T. ) ;
#7009=DIRECTION ( 'NONE',  ( 0.000000000000000000, 1.000000000000000000, 0.000000000000000000 ) ) ;
#7032=ORIENTED_EDGE ( 'NONE', *, *, #8463, .F. ) ;
#7058=FACE_OUTER_BOUND ( 'NONE', #15339, .T. ) ;
#7067=ORIENTED_EDGE ( 'NONE', *, *, #5491, .F. ) ;
#7073=FILL_AREA_STYLE_COLOUR ( '', #10404 ) ;
#7105=ORIENTED_EDGE ( 'NONE', *, *, #808, .F. ) ;
#7120=DIRECTION ( 'NONE',  ( -0.000000000000000000, 1.000000000000000000, -0.000000000000000000 ) ) ;
#7126=AXIS2_PLACEMENT_3D ( 'NONE', #12675, #3696, #11086 ) ;
#7143=DIRECTION ( 'NONE',  ( 0.000000000000000000, 0.000000000000000000, -1.000000000000000000 ) ) ;
#7159=DIRECTION ( 'NONE',  ( 0.000000000000000000, 0.000000000000000000, -1.000000000000000000 ) ) ;
#7162=DIRECTION ( 'NONE',  ( 0.000000000000000000, -1.000000000000000000, 0.000000000000000000 ) ) ;
#7169=CARTESIAN_POINT ( 'NONE',  ( -6.000000000000000000, 24.99999999999999645, -6.000000000000000000 ) ) ;
#7174=EDGE_LOOP ( 'NONE', ( #3910, #16096, #1336, #19890 ) ) ;
#7179=AXIS2_PLACEMENT_3D ( 'NONE', #5985, #8176, #2356 ) ;
#7200=AXIS2_PLACEMENT_3D ( 'NONE', #3190, #10572, #17958 ) ;
#7250=CARTESIAN_POINT ( 'NONE',  ( -4.080056528100000079, 28.00000000000000000, 4.563746053395999702 ) ) ;
#7255=DIRECTION ( 'NONE',  ( 0.000000000000000000, 0.000000000000000000, 1.000000000000000000 ) ) ;
#7257=EDGE_CURVE ( 'NONE', #18186, #18240, #23778, .T. ) ;
#7259=LINE ( 'NONE', #11024, #21951 ) ;
#7280=VERTEX_POINT ( 'NONE', #18452 ) ;
#7284=ORIENTED_EDGE ( 'NONE', *, *, #18849, .T. ) ;
#7317=EDGE_CURVE ( 'NONE', #10530, #9818, #262, .T. ) ;
#7320=ADVANCED_FACE ( 'NONE', ( #13230 ), #9483, .F. ) ;
#7374=EDGE_LOOP ( 'NONE', ( #18554, #4456 ) ) ;
#7410=DIRECTION ( 'NONE',  ( 0.000000000000000000, 0.000000000000000000, 1.000000000000000000 ) ) ;
#7447=DIRECTION ( 'NONE',  ( 0.000000000000000000, -1.000000000000000000, 0.000000000000000000 ) ) ;
#7453=EDGE_LOOP ( 'NONE', ( #6455, #7067, #6937, #20630 ) ) ;
#7504=DIRECTION ( 'NONE',  ( 0.5000000000000169864, -0.8660254037844288266, 0.000000000000000000 ) ) ;
#7515=CARTESIAN_POINT ( 'NONE',  ( -5.204962792833000229, 27.25000000000000000, 2.704962792832999785 ) ) ;
#7520=ORIENTED_EDGE ( 'NONE', *, *, #18603, .F. ) ;
#7533=DIRECTION ( 'NONE',  ( 1.000000000000000000, 0.000000000000000000, 0.000000000000000000 ) ) ;
#7580=VECTOR ( 'NONE', #6094, 1000.000000000000000 ) ;
#7603=AXIS2_PLACEMENT_3D ( 'NONE', #11817, #2241, #19194 ) ;
#7604=CARTESIAN_POINT ( 'NONE',  ( -2.649999999999999911, 28.00000000000000000, 0.000000000000000000 ) ) ;
#7624=( NAMED_UNIT ( * ) PLANE_ANGLE_UNIT ( ) SI_UNIT ( $, .RADIAN. ) );
#7630=EDGE_CURVE ( 'NONE', #14966, #13647, #2963, .T. ) ;
#7644=PLANE ( 'NONE',  #2501 ) ;
#7648=DIRECTION ( 'NONE',  ( 0.000000000000000000, 1.000000000000000000, 0.000000000000000000 ) ) ;
#7649=AXIS2_PLACEMENT_3D ( 'NONE', #424, #9641, #20907 ) ;
#7660=VERTEX_POINT ( 'NONE', #10295 ) ;
#7679=VECTOR ( 'NONE', #17009, 1000.000000000000000 ) ;
#7688=AXIS2_PLACEMENT_3D ( 'NONE', #23178, #6596, #21006 ) ;
#7689=ORIENTED_EDGE ( 'NONE', *, *, #17956, .T. ) ;
#7697=DIRECTION ( 'NONE',  ( 0.000000000000000000, 1.000000000000000000, 0.000000000000000000 ) ) ;
#7734=LINE ( 'NONE', #11012, #21514 ) ;
#7736=DIRECTION ( 'NONE',  ( 0.000000000000000000, 1.000000000000000000, 0.000000000000000000 ) ) ;
#7757=CARTESIAN_POINT ( 'NONE',  ( 22.66677564524290744, 35.31760589360604996, -6.000000000000000000 ) ) ;
#7783=ORIENTED_EDGE ( 'NONE', *, *, #7007, .F. ) ;
#7802=ORIENTED_EDGE ( 'NONE', *, *, #23769, .F. ) ;
#7828=DIRECTION ( 'NONE',  ( 0.000000000000000000, 0.000000000000000000, 1.000000000000000000 ) ) ;
#7843=VECTOR ( 'NONE', #8150, 1000.000000000000000 ) ;
#7876=EDGE_CURVE ( 'NONE', #12335, #9818, #22580, .T. ) ;
#7879=DIRECTION ( 'NONE',  ( 0.000000000000000000, -1.000000000000000000, 0.000000000000000000 ) ) ;
#7884=EDGE_CURVE ( 'NONE', #9739, #15717, #11692, .T. ) ;
#7906=DIRECTION ( 'NONE',  ( 0.000000000000000000, 0.000000000000000000, -1.000000000000000000 ) ) ;
#7909=VECTOR ( 'NONE', #2000, 1000.000000000000000 ) ;
#7916=CARTESIAN_POINT ( 'NONE',  ( 7.446152422707000618, 28.20096189432300093, 6.000000000000000000 ) ) ;
#7937=EDGE_CURVE ( 'NONE', #3633, #11154, #22815, .T. ) ;
#7941=DIRECTION ( 'NONE',  ( 0.000000000000000000, 1.000000000000000000, 0.000000000000000000 ) ) ;
#7943=VERTEX_POINT ( 'NONE', #14944 ) ;
#7963=CARTESIAN_POINT ( 'NONE',  ( -7.500000000000000000, 24.99999999999999645, 1.000000000000000000 ) ) ;
#7969=CARTESIAN_POINT ( 'NONE',  ( 22.66677564524290744, 35.31760589360604996, 6.000000000000000000 ) ) ;
#7972=CARTESIAN_POINT ( 'NONE',  ( 61.60588651278290939, 37.01856778792605240, -1.000000000000000000 ) ) ;
#7975=FACE_OUTER_BOUND ( 'NONE', #9557, .T. ) ;
#7997=CARTESIAN_POINT ( 'NONE',  ( -9.000000000000000000, 18.50000000000000000, -2.000000000000000000 ) ) ;
#8000=DIRECTION ( 'NONE',  ( 0.000000000000000000, 0.000000000000000000, -1.000000000000000000 ) ) ;
#8014=ORIENTED_EDGE ( 'NONE', *, *, #18883, .F. ) ;
#8043=CARTESIAN_POINT ( 'NONE',  ( -7.500000000000000000, 24.99999999999999645, 1.000000000000000000 ) ) ;
#8047=PRODUCT_DEFINITION_SHAPE ( 'NONE', 'NONE',  #5757 ) ;
#8060=STYLED_ITEM ( 'NONE', ( #14457 ), #16570 ) ;
#8076=AXIS2_PLACEMENT_3D ( 'NONE', #20488, #9461, #16835 ) ;
#8095=VECTOR ( 'NONE', #19501, 1000.000000000000114 ) ;
#8096=CARTESIAN_POINT ( 'NONE',  ( -5.730762473771000565, 26.50000000000000000, 1.577381738259000077 ) ) ;
#8118=DIRECTION ( 'NONE',  ( 0.000000000000000000, 0.000000000000000000, -1.000000000000000000 ) ) ;
#8126=LINE ( 'NONE', #7757, #2276 ) ;
#8147=EDGE_CURVE ( 'NONE', #15650, #14474, #4644, .T. ) ;
#8150=DIRECTION ( 'NONE',  ( 1.000000000000000000, 0.000000000000000000, 0.000000000000000000 ) ) ;
#8168=DIRECTION ( 'NONE',  ( 1.000000000000000000, 0.000000000000000000, 0.000000000000000000 ) ) ;
#8176=DIRECTION ( 'NONE',  ( 0.000000000000000000, 0.000000000000000000, 1.000000000000000000 ) ) ;
#8186=ORIENTED_EDGE ( 'NONE', *, *, #19951, .T. ) ;
#8192=CARTESIAN_POINT ( 'NONE',  ( -6.173093822438193712, 26.49020434458659068, 1.113528899897020308 ) ) ;
#8289=DIRECTION ( 'NONE',  ( 0.000000000000000000, 0.000000000000000000, -1.000000000000000000 ) ) ;
#8309=EDGE_CURVE ( 'NONE', #9702, #1360, #16366, .T. ) ;
#8311=CARTESIAN_POINT ( 'NONE',  ( 23.01485185659291233, 35.51856778792605240, 2.673746900119610359 ) ) ;
#8335=DIRECTION ( 'NONE',  ( -1.421085471520000159E-14, 1.000000000000000000, 0.000000000000000000 ) ) ;
#8351=LINE ( 'NONE', #4602, #16318 ) ;
#8384=ADVANCED_FACE ( 'NONE', ( #962 ), #21072, .F. ) ;
#8401=VECTOR ( 'NONE', #17139, 1000.000000000000000 ) ;
#8463=EDGE_CURVE ( 'NONE', #7660, #165, #2012, .T. ) ;
#8465=CIRCLE ( 'NONE', #7179, 1.500000000000001332 ) ;
#8536=DIRECTION ( 'NONE',  ( -0.5000000000000169864, 0.8660254037844288266, 0.000000000000000000 ) ) ;
#8544=EDGE_CURVE ( 'NONE', #9739, #7943, #12244, .T. ) ;
#8552=CARTESIAN_POINT ( 'NONE',  ( -0.7783053373570000266, 26.50000000000000000, 6.000000000000000000 ) ) ;
#8565=ORIENTED_EDGE ( 'NONE', *, *, #8309, .F. ) ;
#8568=DIRECTION ( 'NONE',  ( 0.000000000000000000, 0.000000000000000000, 1.000000000000000000 ) ) ;
#8586=ORIENTED_EDGE ( 'NONE', *, *, #1649, .F. ) ;
#8610=CARTESIAN_POINT ( 'NONE',  ( 61.60588651278290939, 35.51856778792605240, 1.000000000000000000 ) ) ;
#8623=CARTESIAN_POINT ( 'NONE',  ( 22.35132670216743023, 35.07441746931982607, -6.000000000000005329 ) ) ;
#8631=DIRECTION ( 'NONE',  ( -1.000000000000000000, 0.000000000000000000, 0.000000000000000000 ) ) ;
#8686=LINE ( 'NONE', #19830, #4417 ) ;
#8692=DIRECTION ( 'NONE',  ( 0.000000000000000000, -1.000000000000000000, 0.000000000000000000 ) ) ;
#8719=CARTESIAN_POINT ( 'NONE',  ( 23.41677564524290744, 37.01856778792605240, -6.000000000000000000 ) ) ;
#8743=CYLINDRICAL_SURFACE ( 'NONE', #17672, 2.673746900119611247 ) ;
#8755=SHAPE_REPRESENTATION ( 'Flat Lever Handle', ( #4390 ), #11350 ) ;
#8815=CARTESIAN_POINT ( 'NONE',  ( -6.637070260807000466, 26.35799170939839797, 1.000000000000000000 ) ) ;
#8840=ORIENTED_EDGE ( 'NONE', *, *, #10886, .F. ) ;
#8854=DIRECTION ( 'NONE',  ( 1.000000000000000000, 0.000000000000000000, 0.000000000000000000 ) ) ;
#8858=VECTOR ( 'NONE', #289, 1000.000000000000000 ) ;
#8865=AXIS2_PLACEMENT_3D ( 'NONE', #2020, #3841, #5648 ) ;
#8929=DIRECTION ( 'NONE',  ( 0.000000000000000000, 1.000000000000000000, 0.000000000000000000 ) ) ;
#8949=EDGE_CURVE ( 'NONE', #6003, #2681, #1739, .T. ) ;
#8961=CARTESIAN_POINT ( 'NONE',  ( -9.000000000000000000, 18.50000000000000000, -6.000000000000000000 ) ) ;
#8968=DIRECTION ( 'NONE',  ( 0.000000000000000000, 0.000000000000000000, 1.000000000000000000 ) ) ;
#8979=ADVANCED_FACE ( 'NONE', ( #9227 ), #1840, .F. ) ;
#8983=CARTESIAN_POINT ( 'NONE',  ( 0.000000000000000000, 0.000000000000000000, 0.000000000000000000 ) ) ;
#8993=CIRCLE ( 'NONE', #20278, 1.000000000000000000 ) ;
#9000=DIRECTION ( 'NONE',  ( 1.000000000000000000, 0.000000000000000000, 0.000000000000000000 ) ) ;
#9004=EDGE_LOOP ( 'NONE', ( #2318, #399, #21121, #3175 ) ) ;
#9013=VERTEX_POINT ( 'NONE', #12631 ) ;
#9028=DIRECTION ( 'NONE',  ( 0.5000000000000169864, -0.8660254037844289376, 0.000000000000000000 ) ) ;
#9043=CARTESIAN_POINT ( 'NONE',  ( -4.080056528100000079, 28.00000000000000000, 4.563746053395999702 ) ) ;
#9072=ORIENTED_EDGE ( 'NONE', *, *, #19105, .F. ) ;
#9084=CARTESIAN_POINT ( 'NONE',  ( 23.41677564524290744, 34.01856778792605240, 6.000000000000005329 ) ) ;
#9106=ADVANCED_FACE ( 'NONE', ( #22639 ), #7644, .F. ) ;
#9112=EDGE_LOOP ( 'NONE', ( #13628, #14007, #21873, #22493 ) ) ;
#9119=DIRECTION ( 'NONE',  ( 0.000000000000000000, 0.000000000000000000, -1.000000000000000000 ) ) ;
#9136=B_SPLINE_CURVE_WITH_KNOTS ( 'NONE', 3,
 ( #18847, #15319, #22710, #8192, #2620, #20910, #15561, #5774, #2136, #9525 ),
 .UNSPECIFIED., .F., .F.,
 ( 4, 2, 2, 2, 4 ),
 ( 0.000000000000000000, 0.2500000000000002220, 0.3750000000000003331, 0.5000000000000004441, 1.000000000000000000 ),
 .UNSPECIFIED. ) ;
#9139=ORIENTED_EDGE ( 'NONE', *, *, #583, .T. ) ;
#9166=ORIENTED_EDGE ( 'NONE', *, *, #7884, .T. ) ;
#9179=EDGE_LOOP ( 'NONE', ( #11537, #19346, #21203, #3359 ) ) ;
#9187=PLANE ( 'NONE',  #412 ) ;
#9191=CARTESIAN_POINT ( 'NONE',  ( -7.500000000000000000, 26.50000000000000000, -6.000000000000000000 ) ) ;
#9227=FACE_OUTER_BOUND ( 'NONE', #21737, .T. ) ;
#9249=CARTESIAN_POINT ( 'NONE',  ( 23.41677564524290744, 34.01856778792605240, -6.000000000000000000 ) ) ;
#9250=CARTESIAN_POINT ( 'NONE',  ( 23.41677564524290744, 35.51856778792605240, -6.000000000000000000 ) ) ;
#9266=DIRECTION ( 'NONE',  ( -0.2123567536025093572, 0.9771922068863437838, 0.000000000000000000 ) ) ;
#9281=LINE ( 'NONE', #6987, #1905 ) ;
#9283=ADVANCED_FACE ( 'NONE', ( #22883 ), #4365, .T. ) ;
#9289=ORIENTED_EDGE ( 'NONE', *, *, #7630, .F. ) ;
#9333=LINE ( 'NONE', #17186, #13223 ) ;
#9334=ORIENTED_EDGE ( 'NONE', *, *, #20798, .F. ) ;
#9367=VECTOR ( 'NONE', #10685, 1000.000000000000000 ) ;
#9384=AXIS2_PLACEMENT_3D ( 'NONE', #3996, #15115, #4 ) ;
#9393=FACE_OUTER_BOUND ( 'NONE', #4774, .T. ) ;
#9419=CARTESIAN_POINT ( 'NONE',  ( -9.000000000000000000, 19.50000000000000000, -6.000000000000000000 ) ) ;
#9426=DIRECTION ( 'NONE',  ( -1.000000000000000000, 0.000000000000000000, 0.000000000000000000 ) ) ;
#9428=DIRECTION ( 'NONE',  ( 0.000000000000000000, 0.000000000000000000, -1.000000000000000000 ) ) ;
#9431=ORIENTED_EDGE ( 'NONE', *, *, #13521, .T. ) ;
#9461=DIRECTION ( 'NONE',  ( 0.000000000000000000, 1.000000000000000000, 0.000000000000000000 ) ) ;
#9483=PLANE ( 'NONE',  #6807 ) ;
#9510=DIRECTION ( 'NONE',  ( 0.000000000000000000, 0.000000000000000000, 1.000000000000000000 ) ) ;
#9511=CYLINDRICAL_SURFACE ( 'NONE', #18158, 1.000000000000000222 ) ;
#9525=CARTESIAN_POINT ( 'NONE',  ( -6.637070260807000466, 26.35799170939839797, 1.000000000000000000 ) ) ;
#9527=ADVANCED_FACE ( 'NONE', ( #15787 ), #2968, .F. ) ;
#9532=VERTEX_POINT ( 'NONE', #6348 ) ;
#9554=EDGE_LOOP ( 'NONE', ( #10911, #11379, #3937, #23562 ) ) ;
#9555=CIRCLE ( 'NONE', #15733, 2.649999999999999911 ) ;
#9557=EDGE_LOOP ( 'NONE', ( #15386, #17619, #5529, #18525, #23281, #677, #21990, #5313 ) ) ;
#9577=DIRECTION ( 'NONE',  ( 0.000000000000000000, -1.000000000000000000, 0.000000000000000000 ) ) ;
#9586=LINE ( 'NONE', #13214, #3854 ) ;
#9587=CARTESIAN_POINT ( 'NONE',  ( -0.7783053373570000266, 28.00000000000000000, 6.000000000000000000 ) ) ;
#9641=DIRECTION ( 'NONE',  ( 0.000000000000000000, 0.000000000000000000, -1.000000000000000000 ) ) ;
#9643=EDGE_CURVE ( 'NONE', #9739, #11734, #3459, .T. ) ;
#9656=DIRECTION ( 'NONE',  ( 0.000000000000000000, 0.000000000000000000, 1.000000000000000000 ) ) ;
#9671=CARTESIAN_POINT ( 'NONE',  ( 0.000000000000000000, 27.25000000000000000, 0.000000000000000000 ) ) ;
#9676=EDGE_LOOP ( 'NONE', ( #823, #5843, #7689, #12114 ) ) ;
#9700=EDGE_CURVE ( 'NONE', #11090, #4666, #16212, .T. ) ;
#9702=VERTEX_POINT ( 'NONE', #19747 ) ;
#9739=VERTEX_POINT ( 'NONE', #8719 ) ;
#9741=LINE ( 'NONE', #13252, #7580 ) ;
#9742=CIRCLE ( 'NONE', #18263, 2.999999999999999556 ) ;
#9744=DIRECTION ( 'NONE',  ( 0.000000000000000000, 0.000000000000000000, 1.000000000000000000 ) ) ;
#9753=CARTESIAN_POINT ( 'NONE',  ( -0.7783053373570000266, 26.50000000000000000, 6.000000000000000000 ) ) ;
#9777=AXIS2_PLACEMENT_3D ( 'NONE', #10083, #10328, #4639 ) ;
#9781=ORIENTED_EDGE ( 'NONE', *, *, #1541, .T. ) ;
#9815=VECTOR ( 'NONE', #736, 1000.000000000000114 ) ;
#9818=VERTEX_POINT ( 'NONE', #20323 ) ;
#9847=ADVANCED_FACE ( 'NONE', ( #5319 ), #20102, .T. ) ;
#9850=EDGE_CURVE ( 'NONE', #12335, #23570, #18279, .T. ) ;
#9857=DIRECTION ( 'NONE',  ( 0.000000000000000000, 1.000000000000000000, 0.000000000000000000 ) ) ;
#9862=VERTEX_POINT ( 'NONE', #13280 ) ;
#9897=AXIS2_PLACEMENT_3D ( 'NONE', #12937, #20567, #18746 ) ;
#9947=ORIENTED_EDGE ( 'NONE', *, *, #16757, .T. ) ;
#9971=VERTEX_POINT ( 'NONE', #1546 ) ;
#9980=CARTESIAN_POINT ( 'NONE',  ( 8.196152422706999729, 26.90192378864669820, -6.000000000000000000 ) ) ;
#10009=DIRECTION ( 'NONE',  ( 0.000000000000000000, 1.000000000000000000, 0.000000000000000000 ) ) ;
#10046=CARTESIAN_POINT ( 'NONE',  ( -8.250000000000000000, 22.00000000000000000, 2.500000000000000000 ) ) ;
#10053=DIRECTION ( 'NONE',  ( -1.000000000000000000, 0.000000000000000000, 0.000000000000000000 ) ) ;
#10064=DIRECTION ( 'NONE',  ( -0.000000000000000000, 1.000000000000000000, 0.000000000000000000 ) ) ;
#10083=CARTESIAN_POINT ( 'NONE',  ( 0.000000000000000000, 28.00000000000000000, 0.000000000000000000 ) ) ;
#10092=ORIENTED_EDGE ( 'NONE', *, *, #17257, .F. ) ;
#10118=CARTESIAN_POINT ( 'NONE',  ( 23.41677564524290744, 37.01856778792605240, 6.000000000000000000 ) ) ;
#10159=EDGE_CURVE ( 'NONE', #15280, #22896, #9586, .T. ) ;
#10186=LINE ( 'NONE', #10307, #3477 ) ;
#10191=DIRECTION ( 'NONE',  ( 0.9063077870366026412, 0.000000000000000000, -0.4226182617408008602 ) ) ;
#10285=VECTOR ( 'NONE', #5847, 1000.000000000000000 ) ;
#10295=CARTESIAN_POINT ( 'NONE',  ( 30.87226923053214378, 35.51856778792605240, 2.673746900119611247 ) ) ;
#10297=VERTEX_POINT ( 'NONE', #1847 ) ;
#10307=CARTESIAN_POINT ( 'NONE',  ( 61.60588651278290939, 37.01856778792605240, 6.000000000000000000 ) ) ;
#10318=LINE ( 'NONE', #2688, #9815 ) ;
#10328=DIRECTION ( 'NONE',  ( 0.000000000000000000, 1.000000000000000000, 0.000000000000000000 ) ) ;
#10339=VERTEX_POINT ( 'NONE', #5306 ) ;
#10346=DIRECTION ( 'NONE',  ( 0.000000000000000000, 0.000000000000000000, -1.000000000000000000 ) ) ;
#10368=ORIENTED_EDGE ( 'NONE', *, *, #13234, .F. ) ;
#10400=LINE ( 'NONE', #14147, #21997 ) ;
#10404=COLOUR_RGB ( '', 0.72549020, 0.75294118, 0.79215686) ;
#10410=DIRECTION ( 'NONE',  ( 0.000000000000000000, -1.000000000000000000, 0.000000000000000000 ) ) ;
#10412=CARTESIAN_POINT ( 'NONE',  ( 6.696152422707000618, 28.00000000000000000, 6.000000000000000000 ) ) ;
#10459=EDGE_CURVE ( 'NONE', #15241, #20808, #22027, .T. ) ;
#10467=ORIENTED_EDGE ( 'NONE', *, *, #20180, .F. ) ;
#10517=FACE_OUTER_BOUND ( 'NONE', #19668, .T. ) ;
#10520=CARTESIAN_POINT ( 'NONE',  ( -7.500000000000000000, 19.50000000000000000, -2.000000000000000000 ) ) ;
#10530=VERTEX_POINT ( 'NONE', #15080 ) ;
#10566=ORIENTED_EDGE ( 'NONE', *, *, #20786, .T. ) ;
#10572=DIRECTION ( 'NONE',  ( 0.000000000000000000, 1.000000000000000000, 0.000000000000000000 ) ) ;
#10581=CARTESIAN_POINT ( 'NONE',  ( -8.250000000000000000, 20.24999999999999645, -1.000000000000000000 ) ) ;
#10585=ADVANCED_FACE ( 'NONE', ( #793 ), #427, .T. ) ;
#10594=EDGE_CURVE ( 'NONE', #2374, #13175, #9136, .T. ) ;
#10599=EDGE_LOOP ( 'NONE', ( #7802, #1449, #20079, #10566, #22215, #19137 ) ) ;
#10603=VECTOR ( 'NONE', #5866, 1000.000000000000000 ) ;
#10617=DIRECTION ( 'NONE',  ( 0.000000000000000000, 0.000000000000000000, -1.000000000000000000 ) ) ;
#10623=AXIS2_PLACEMENT_3D ( 'NONE', #5977, #8168, #2350 ) ;
#10625=CARTESIAN_POINT ( 'NONE',  ( 22.83443279375291368, 36.19190089707605296, -6.000000000000000000 ) ) ;
#10636=DIRECTION ( 'NONE',  ( 0.000000000000000000, 0.000000000000000000, 1.000000000000000000 ) ) ;
#10683=ORIENTED_EDGE ( 'NONE', *, *, #15585, .F. ) ;
#10685=DIRECTION ( 'NONE',  ( -0.000000000000000000, 1.000000000000000000, -0.000000000000000000 ) ) ;
#10737=EDGE_CURVE ( 'NONE', #3633, #11775, #20450, .T. ) ;
#10758=CARTESIAN_POINT ( 'NONE',  ( 0.000000000000000000, 26.50000000000000000, 0.000000000000000000 ) ) ;
#10794=ORIENTED_EDGE ( 'NONE', *, *, #10459, .T. ) ;
#10795=CARTESIAN_POINT ( 'NONE',  ( 23.41677564524290744, 35.51856778792605240, -6.000000000000000000 ) ) ;
#10802=DIRECTION ( 'NONE',  ( -0.000000000000000000, 1.000000000000000000, -0.000000000000000000 ) ) ;
#10810=CARTESIAN_POINT ( 'NONE',  ( 30.87226923053214378, 27.01856778792605240, 2.673746900119611247 ) ) ;
#10816=AXIS2_PLACEMENT_3D ( 'NONE', #19204, #6492, #13875 ) ;
#10817=DIRECTION ( 'NONE',  ( 1.000000000000000000, 0.000000000000000000, 0.000000000000000000 ) ) ;
#10827=CIRCLE ( 'NONE', #734, 1.000000000000000000 ) ;
#10831=CARTESIAN_POINT ( 'NONE',  ( -6.000000000000000000, 24.99999999999999645, -6.000000000000000000 ) ) ;
#10840=EDGE_LOOP ( 'NONE', ( #728, #16230, #3860, #20006 ) ) ;
#10850=ORIENTED_EDGE ( 'NONE', *, *, #19473, .T. ) ;
#10867=CARTESIAN_POINT ( 'NONE',  ( 6.696152422707000618, 28.00000000000000000, -6.000000000000000000 ) ) ;
#10886=EDGE_CURVE ( 'NONE', #11418, #19500, #3407, .T. ) ;
#10889=LINE ( 'NONE', #12703, #311 ) ;
#10892=UNCERTAINTY_MEASURE_WITH_UNIT (LENGTH_MEASURE( 1.000000000000000082E-05 ), #22052, 'distance_accuracy_value', 'NONE');
#10893=DIRECTION ( 'NONE',  ( 0.000000000000000000, -1.000000000000000000, 0.000000000000000000 ) ) ;
#10898=CARTESIAN_POINT ( 'NONE',  ( 61.60588651278290939, 37.01856778792605240, 1.000000000000000000 ) ) ;
#10911=ORIENTED_EDGE ( 'NONE', *, *, #3708, .T. ) ;
#10916=CIRCLE ( 'NONE', #23276, 2.999999999999999112 ) ;
#10943=ORIENTED_EDGE ( 'NONE', *, *, #1977, .F. ) ;
#10946=DIRECTION ( 'NONE',  ( 0.000000000000000000, 0.000000000000000000, 1.000000000000000000 ) ) ;
#10998=CARTESIAN_POINT ( 'NONE',  ( 60.61494135913342518, 27.01856778792605240, 0.000000000000000000 ) ) ;
#11012=CARTESIAN_POINT ( 'NONE',  ( -5.730762473771000565, 26.50000000000000000, 1.577381738259000077 ) ) ;
#11020=CARTESIAN_POINT ( 'NONE',  ( 66.60588651278291650, 35.51856778792605240, -1.000000000000000000 ) ) ;
#11024=CARTESIAN_POINT ( 'NONE',  ( 6.696152422707000618, 28.00000000000000000, 6.000000000000000000 ) ) ;
#11030=ORIENTED_EDGE ( 'NONE', *, *, #8309, .T. ) ;
#11054=CARTESIAN_POINT ( 'NONE',  ( 6.696152422707000618, 29.50000000000000000, -6.000000000000000000 ) ) ;
#11056=DIRECTION ( 'NONE',  ( -1.000000000000000000, -0.000000000000000000, -0.000000000000000000 ) ) ;
#11086=DIRECTION ( 'NONE',  ( 1.561251128379125123E-14, -1.000000000000000000, 0.000000000000000000 ) ) ;
#11087=B_SPLINE_CURVE_WITH_KNOTS ( 'NONE', 3,
 ( #11980, #22858, #6272, #21302 ),
 .UNSPECIFIED., .F., .F.,
 ( 4, 4 ),
 ( 0.000000000000000000, 1.000000000000000000 ),
 .UNSPECIFIED. ) ;
#11090=VERTEX_POINT ( 'NONE', #7969 ) ;
#11096=DIRECTION ( 'NONE',  ( 0.000000000000000000, 0.000000000000000000, 1.000000000000000000 ) ) ;
#11111=ORIENTED_EDGE ( 'NONE', *, *, #12035, .F. ) ;
#11137=EDGE_LOOP ( 'NONE', ( #13820, #5396, #5864, #20256, #17564, #22859, #20181, #6631 ) ) ;
#11138=CARTESIAN_POINT ( 'NONE',  ( 66.60588651278291650, 35.51856778792605240, -1.000000000000000000 ) ) ;
#11148=EDGE_LOOP ( 'NONE', ( #20333, #15624, #14071, #7032 ) ) ;
#11151=VECTOR ( 'NONE', #8854, 1000.000000000000000 ) ;
#11154=VERTEX_POINT ( 'NONE', #7604 ) ;
#11164=AXIS2_PLACEMENT_3D ( 'NONE', #10831, #18217, #1619 ) ;
#11171=ORIENTED_EDGE ( 'NONE', *, *, #8544, .F. ) ;
#11182=ORIENTED_EDGE ( 'NONE', *, *, #23501, .F. ) ;
#11201=ORIENTED_EDGE ( 'NONE', *, *, #13356, .T. ) ;
#11239=EDGE_LOOP ( 'NONE', ( #22993, #6424, #10683, #6846 ) ) ;
#11243=ORIENTED_EDGE ( 'NONE', *, *, #502, .F. ) ;
#11276=FACE_OUTER_BOUND ( 'NONE', #21024, .T. ) ;
#11291=DIRECTION ( 'NONE',  ( 0.000000000000000000, 0.000000000000000000, 1.000000000000000000 ) ) ;
#11299=DIRECTION ( 'NONE',  ( 0.000000000000000000, -1.000000000000000000, 0.000000000000000000 ) ) ;
#11311=CARTESIAN_POINT ( 'NONE',  ( 21.45754691133435799, 36.29044427405532502, -115.0195023120000002 ) ) ;
#11350=( GEOMETRIC_REPRESENTATION_CONTEXT ( 3 ) GLOBAL_UNCERTAINTY_ASSIGNED_CONTEXT ( ( #10892 ) ) GLOBAL_UNIT_ASSIGNED_CONTEXT ( ( #22052, #7624, #18534 ) ) REPRESENTATION_CONTEXT ( 'NONE', 'WORKASPACE' ) );
#11354=CARTESIAN_POINT ( 'NONE',  ( -6.000000000000000000, 24.99999999999999645, -115.0195023120000002 ) ) ;
#11367=AXIS2_PLACEMENT_3D ( 'NONE', #4411, #11449, #20762 ) ;
#11379=ORIENTED_EDGE ( 'NONE', *, *, #9850, .T. ) ;
#11418=VERTEX_POINT ( 'NONE', #20905 ) ;
#11430=ADVANCED_FACE ( 'NONE', ( #13028 ), #5767, .F. ) ;
#11438=VERTEX_POINT ( 'NONE', #22704 ) ;
#11449=DIRECTION ( 'NONE',  ( 0.000000000000000000, -1.000000000000000000, 0.000000000000000000 ) ) ;
#11450=ORIENTED_EDGE ( 'NONE', *, *, #19897, .T. ) ;
#11534=LINE ( 'NONE', #5944, #11760 ) ;
#11537=ORIENTED_EDGE ( 'NONE', *, *, #7257, .F. ) ;
#11560=VECTOR ( 'NONE', #6214, 1000.000000000000000 ) ;
#11562=EDGE_CURVE ( 'NONE', #9013, #611, #15249, .T. ) ;
#11565=DIRECTION ( 'NONE',  ( 0.000000000000000000, -1.000000000000000000, 0.000000000000000000 ) ) ;
#11569=CARTESIAN_POINT ( 'NONE',  ( -0.7783053373570000266, 84.95442836047000412, 5.000000000000000000 ) ) ;
#11570=CYLINDRICAL_SURFACE ( 'NONE', #17086, 1.000000000000000222 ) ;
#11573=AXIS2_PLACEMENT_3D ( 'NONE', #17782, #1301, #8692 ) ;
#11587=AXIS2_PLACEMENT_3D ( 'NONE', #22829, #20788, #2373 ) ;
#11642=LINE ( 'NONE', #7997, #2529 ) ;
#11656=ORIENTED_EDGE ( 'NONE', *, *, #3772, .F. ) ;
#11667=LINE ( 'NONE', #506, #22218 ) ;
#11679=CARTESIAN_POINT ( 'NONE',  ( -9.000000000000000000, 19.50000000000000000, -1.000000000000000000 ) ) ;
#11684=VECTOR ( 'NONE', #8929, 1000.000000000000000 ) ;
#11692=LINE ( 'NONE', #20651, #23826 ) ;
#11696=LINE ( 'NONE', #18714, #12655 ) ;
#11702=DIRECTION ( 'NONE',  ( 1.000000000000000000, 0.000000000000000000, 0.000000000000000000 ) ) ;
#11710=EDGE_CURVE ( 'NONE', #2875, #9862, #22777, .T. ) ;
#11721=CIRCLE ( 'NONE', #9777, 2.649999999999999911 ) ;
#11725=LINE ( 'NONE', #8096, #16194 ) ;
#11734=VERTEX_POINT ( 'NONE', #23731 ) ;
#11760=VECTOR ( 'NONE', #11056, 1000.000000000000000 ) ;
#11775=VERTEX_POINT ( 'NONE', #14527 ) ;
#11781=LINE ( 'NONE', #13704, #7843 ) ;
#11817=CARTESIAN_POINT ( 'NONE',  ( 66.60588651278291650, 36.26856778792605240, 0.000000000000000000 ) ) ;
#11834=ORIENTED_EDGE ( 'NONE', *, *, #15602, .F. ) ;
#11844=CARTESIAN_POINT ( 'NONE',  ( -4.563746053395999702, 26.50000000000000000, 4.080056528100000079 ) ) ;
#11846=CARTESIAN_POINT ( 'NONE',  ( 8.196152422706999729, 26.90192378864669820, 6.000000000000000000 ) ) ;
#11873=CARTESIAN_POINT ( 'NONE',  ( 0.000000000000000000, 27.25000000000000000, 0.000000000000000000 ) ) ;
#11877=VECTOR ( 'NONE', #8536, 1000.000000000000114 ) ;
#11891=EDGE_CURVE ( 'NONE', #20808, #7660, #2616, .T. ) ;
#11980=CARTESIAN_POINT ( 'NONE',  ( -6.637070260807000466, 27.93157662065900126, 1.000000000000000000 ) ) ;
#12014=CARTESIAN_POINT ( 'NONE',  ( 23.41677564524290744, 34.01856778792605240, 6.000000000000000000 ) ) ;
#12020=ADVANCED_FACE ( 'NONE', ( #17397 ), #21638, .T. ) ;
#12035=EDGE_CURVE ( 'NONE', #16279, #13125, #20861, .T. ) ;
#12040=VECTOR ( 'NONE', #5321, 1000.000000000000000 ) ;
#12052=CYLINDRICAL_SURFACE ( 'NONE', #5741, 1.000000000000000000 ) ;
#12077=VECTOR ( 'NONE', #732, 1000.000000000000000 ) ;
#12114=ORIENTED_EDGE ( 'NONE', *, *, #11710, .F. ) ;
#12133=DIRECTION ( 'NONE',  ( 1.000000000000000000, 0.000000000000000000, 0.000000000000000000 ) ) ;
#12160=DIRECTION ( 'NONE',  ( 0.000000000000000000, 1.000000000000000000, 0.000000000000000000 ) ) ;
#12178=VECTOR ( 'NONE', #8631, 1000.000000000000000 ) ;
#12188=AXIS2_PLACEMENT_3D ( 'NONE', #21834, #9000, #21723 ) ;
#12222=CARTESIAN_POINT ( 'NONE',  ( -7.500000000000000000, 28.00000000000000000, -6.000000000000000000 ) ) ;
#12224=LINE ( 'NONE', #21306, #16901 ) ;
#12227=EDGE_CURVE ( 'NONE', #19197, #11438, #6084, .T. ) ;
#12232=CIRCLE ( 'NONE', #6422, 2.999999999999999112 ) ;
#12244=LINE ( 'NONE', #1459, #11151 ) ;
#12272=DIRECTION ( 'NONE',  ( -1.000000000000000000, 0.000000000000000000, -0.000000000000000000 ) ) ;
#12283=LINE ( 'NONE', #19673, #19581 ) ;
#12289=EDGE_LOOP ( 'NONE', ( #17289, #6121, #20738, #6692, #12660, #16174, #230, #8186, #20668 ) ) ;
#12293=EDGE_LOOP ( 'NONE', ( #13569, #22528, #5287, #22418, #22559, #22885 ) ) ;
#12318=ORIENTED_EDGE ( 'NONE', *, *, #17065, .F. ) ;
#12319=DIRECTION ( 'NONE',  ( -0.000000000000000000, 1.000000000000000000, -0.000000000000000000 ) ) ;
#12335=VERTEX_POINT ( 'NONE', #7916 ) ;
#12343=AXIS2_PLACEMENT_3D ( 'NONE', #7972, #17294, #1061 ) ;
#12344=( GEOMETRIC_REPRESENTATION_CONTEXT ( 3 ) GLOBAL_UNCERTAINTY_ASSIGNED_CONTEXT ( ( #20100 ) ) GLOBAL_UNIT_ASSIGNED_CONTEXT ( ( #6831, #23544, #3455 ) ) REPRESENTATION_CONTEXT ( 'NONE', 'WORKASPACE' ) );
#12406=DIRECTION ( 'NONE',  ( 0.000000000000000000, 0.000000000000000000, 1.000000000000000000 ) ) ;
#12463=DIRECTION ( 'NONE',  ( 0.000000000000000000, -1.000000000000000000, 0.000000000000000000 ) ) ;
#12509=LINE ( 'NONE', #21597, #12178 ) ;
#12522=DIRECTION ( 'NONE',  ( 0.000000000000000000, 1.000000000000000000, 0.000000000000000000 ) ) ;
#12529=DIRECTION ( 'NONE',  ( 0.000000000000000000, 1.000000000000000000, 0.000000000000000000 ) ) ;
#12542=EDGE_CURVE ( 'NONE', #5263, #165, #15782, .T. ) ;
#12548=AXIS2_PLACEMENT_3D ( 'NONE', #4676, #7410, #5717 ) ;
#12555=VERTEX_POINT ( 'NONE', #20722 ) ;
#12590=ORIENTED_EDGE ( 'NONE', *, *, #208, .F. ) ;
#12595=CIRCLE ( 'NONE', #23398, 2.649999999999999911 ) ;
#12601=CARTESIAN_POINT ( 'NONE',  ( 7.278495274186999708, 27.32666689084959799, -6.000000000000000000 ) ) ;
#12605=CARTESIAN_POINT ( 'NONE',  ( -9.000000000000000000, 18.50000000000000000, -5.000000000000000000 ) ) ;
#12631=CARTESIAN_POINT ( 'NONE',  ( -9.000000000000000000, 22.00000000000000000, 1.000000000000000000 ) ) ;
#12647=ORIENTED_EDGE ( 'NONE', *, *, #4688, .T. ) ;
#12655=VECTOR ( 'NONE', #7941, 1000.000000000000000 ) ;
#12660=ORIENTED_EDGE ( 'NONE', *, *, #634, .F. ) ;
#12675=CARTESIAN_POINT ( 'NONE',  ( 6.696152422707000618, 29.50000000000000000, 6.000000000000000000 ) ) ;
#12703=CARTESIAN_POINT ( 'NONE',  ( 2.649999999999999911, 26.50000000000000000, 0.000000000000000000 ) ) ;
#12725=ORIENTED_EDGE ( 'NONE', *, *, #23121, .F. ) ;
#12736=DIRECTION ( 'NONE',  ( -0.000000000000000000, 0.000000000000000000, 1.000000000000000000 ) ) ;
#12745=CARTESIAN_POINT ( 'NONE',  ( 6.696152422707000618, 26.50000000000000000, 6.000000000000000000 ) ) ;
#12766=AXIS2_PLACEMENT_3D ( 'NONE', #11354, #7828, #10009 ) ;
#12784=EDGE_CURVE ( 'NONE', #9532, #11090, #16559, .T. ) ;
#12790=EDGE_CURVE ( 'NONE', #13009, #2875, #19876, .T. ) ;
#12809=LINE ( 'NONE', #637, #11560 ) ;
#12817=LINE ( 'NONE', #18168, #8858 ) ;
#12838=ORIENTED_EDGE ( 'NONE', *, *, #16152, .T. ) ;
#12852=DIRECTION ( 'NONE',  ( 0.000000000000000000, 0.000000000000000000, -1.000000000000000000 ) ) ;
#12923=CYLINDRICAL_SURFACE ( 'NONE', #2603, 1.500000000000001332 ) ;
#12937=CARTESIAN_POINT ( 'NONE',  ( 23.01485185659291233, 35.51856778792605240, -6.000000000000000000 ) ) ;
#12965=CARTESIAN_POINT ( 'NONE',  ( 30.87226923053214378, 35.51856778792605240, 0.000000000000000000 ) ) ;
#13003=VERTEX_POINT ( 'NONE', #16695 ) ;
#13009=VERTEX_POINT ( 'NONE', #11138 ) ;
#13028=FACE_OUTER_BOUND ( 'NONE', #9554, .T. ) ;
#13051=CIRCLE ( 'NONE', #22333, 1.499999999999999778 ) ;
#13102=VECTOR ( 'NONE', #17160, 1000.000000000000000 ) ;
#13104=PLANE ( 'NONE',  #14473 ) ;
#13125=VERTEX_POINT ( 'NONE', #22737 ) ;
#13159=ORIENTED_EDGE ( 'NONE', *, *, #12784, .T. ) ;
#13175=VERTEX_POINT ( 'NONE', #2399 ) ;
#13190=DIRECTION ( 'NONE',  ( -1.000000000000000000, -2.775557561562888827E-14, 0.000000000000000000 ) ) ;
#13211=ADVANCED_FACE ( 'NONE', ( #7975 ), #4589, .T. ) ;
#13214=CARTESIAN_POINT ( 'NONE',  ( -6.000000000000000000, 28.00000000000000000, -6.000000000000000000 ) ) ;
#13220=ORIENTED_EDGE ( 'NONE', *, *, #5912, .T. ) ;
#13223=VECTOR ( 'NONE', #229, 1000.000000000000114 ) ;
#13228=CARTESIAN_POINT ( 'NONE',  ( -7.500000000000000000, 19.50000000000000000, -1.000000000000000000 ) ) ;
#13230=FACE_OUTER_BOUND ( 'NONE', #16798, .T. ) ;
#13234=EDGE_CURVE ( 'NONE', #16279, #22896, #11087, .T. ) ;
#13252=CARTESIAN_POINT ( 'NONE',  ( -6.000000000000000000, 28.00000000000000000, -6.000000000000000000 ) ) ;
#13261=EDGE_CURVE ( 'NONE', #18177, #19500, #20439, .T. ) ;
#13280=CARTESIAN_POINT ( 'NONE',  ( 61.60588651278290939, 35.51856778792605240, 6.000000000000000000 ) ) ;
#13296=VERTEX_POINT ( 'NONE', #18615 ) ;
#13338=DIRECTION ( 'NONE',  ( 0.000000000000000000, 0.000000000000000000, 1.000000000000000000 ) ) ;
#13356=EDGE_CURVE ( 'NONE', #18186, #23810, #12809, .T. ) ;
#13360=LINE ( 'NONE', #8043, #20666 ) ;
#13378=EDGE_CURVE ( 'NONE', #9702, #3316, #17976, .T. ) ;
#13411=AXIS2_PLACEMENT_3D ( 'NONE', #14998, #5808, #13190 ) ;
#13428=ORIENTED_EDGE ( 'NONE', *, *, #4688, .F. ) ;
#13449=LINE ( 'NONE', #13689, #15136 ) ;
#13452=CARTESIAN_POINT ( 'NONE',  ( -7.500000000000000000, 19.50000000000000000, -6.000000000000000000 ) ) ;
#13466=AXIS2_PLACEMENT_3D ( 'NONE', #4258, #7648, #11291 ) ;
#13469=CARTESIAN_POINT ( 'NONE',  ( 30.87226923053214378, 37.01856778792605240, 2.673746900119611247 ) ) ;
#13485=CARTESIAN_POINT ( 'NONE',  ( -9.000000000000000000, 22.00000000000000000, -1.000000000000000000 ) ) ;
#13493=VECTOR ( 'NONE', #11096, 1000.000000000000000 ) ;
#13519=EDGE_CURVE ( 'NONE', #23889, #1360, #6524, .T. ) ;
#13521=EDGE_CURVE ( 'NONE', #21343, #2374, #3555, .T. ) ;
#13540=DIRECTION ( 'NONE',  ( 0.000000000000000000, 1.000000000000000000, 0.000000000000000000 ) ) ;
#13548=EDGE_CURVE ( 'NONE', #21343, #19197, #2262, .T. ) ;
#13557=ORIENTED_EDGE ( 'NONE', *, *, #12542, .F. ) ;
#13569=ORIENTED_EDGE ( 'NONE', *, *, #9643, .T. ) ;
#13574=DIRECTION ( 'NONE',  ( 0.000000000000000000, 0.000000000000000000, -1.000000000000000000 ) ) ;
#13577=CARTESIAN_POINT ( 'NONE',  ( 23.41677564524290744, 35.51856778792605240, 6.000000000000000000 ) ) ;
#13607=LINE ( 'NONE', #4416, #4332 ) ;
#13616=FACE_OUTER_BOUND ( 'NONE', #16826, .T. ) ;
#13623=ADVANCED_FACE ( 'NONE', ( #22535, #4132 ), #371, .F. ) ;
#13628=ORIENTED_EDGE ( 'NONE', *, *, #7937, .T. ) ;
#13642=VECTOR ( 'NONE', #20971, 1000.000000000000000 ) ;
#13646=DIRECTION ( 'NONE',  ( 1.184237892933000067E-14, 1.000000000000000000, 2.412884706852000360E-14 ) ) ;
#13647=VERTEX_POINT ( 'NONE', #9587 ) ;
#13662=CARTESIAN_POINT ( 'NONE',  ( -1.200923599098000061, 28.00000000000000000, 5.906307787036999990 ) ) ;
#13689=CARTESIAN_POINT ( 'NONE',  ( -6.000000000000000000, 26.50000000000000000, -6.000000000000000000 ) ) ;
#13703=ORIENTED_EDGE ( 'NONE', *, *, #5131, .F. ) ;
#13704=CARTESIAN_POINT ( 'NONE',  ( 23.01485185659291233, 35.51856778792605240, -2.673746900119611247 ) ) ;
#13729=DIRECTION ( 'NONE',  ( 0.000000000000000000, -1.000000000000000000, 0.000000000000000000 ) ) ;
#13817=DIRECTION ( 'NONE',  ( 0.000000000000000000, 0.000000000000000000, 1.000000000000000000 ) ) ;
#13820=ORIENTED_EDGE ( 'NONE', *, *, #8147, .T. ) ;
#13837=EDGE_CURVE ( 'NONE', #3316, #17036, #7259, .T. ) ;
#13863=AXIS2_PLACEMENT_3D ( 'NONE', #15064, #19854, #3270 ) ;
#13873=AXIS2_PLACEMENT_3D ( 'NONE', #13903, #6153, #13540 ) ;
#13875=DIRECTION ( 'NONE',  ( 0.000000000000000000, 1.000000000000000000, 0.000000000000000000 ) ) ;
#13903=CARTESIAN_POINT ( 'NONE',  ( -7.500000000000000000, 18.50000000000000000, -6.000000000000000000 ) ) ;
#13939=CARTESIAN_POINT ( 'NONE',  ( -6.637070260807000466, 26.50000000000000000, 2.000000000000000000 ) ) ;
#13977=ORIENTED_EDGE ( 'NONE', *, *, #1276, .F. ) ;
#14005=CARTESIAN_POINT ( 'NONE',  ( 30.87226923053214378, 37.01856778792605240, 2.673746900119610359 ) ) ;
#14007=ORIENTED_EDGE ( 'NONE', *, *, #23501, .T. ) ;
#14024=VECTOR ( 'NONE', #2205, 1000.000000000000000 ) ;
#14033=CARTESIAN_POINT ( 'NONE',  ( 66.60588651278291650, 37.01856778792605240, 1.000000000000000000 ) ) ;
#14059=ORIENTED_EDGE ( 'NONE', *, *, #3593, .F. ) ;
#14071=ORIENTED_EDGE ( 'NONE', *, *, #12542, .T. ) ;
#14083=VERTEX_POINT ( 'NONE', #14033 ) ;
#14097=ORIENTED_EDGE ( 'NONE', *, *, #1541, .F. ) ;
#14111=EDGE_LOOP ( 'NONE', ( #4650, #14389, #11111, #22053, #2914 ) ) ;
#14134=EDGE_CURVE ( 'NONE', #13647, #3316, #12224, .T. ) ;
#14137=ADVANCED_FACE ( 'NONE', ( #23345 ), #2899, .T. ) ;
#14142=ORIENTED_EDGE ( 'NONE', *, *, #15163, .F. ) ;
#14147=CARTESIAN_POINT ( 'NONE',  ( 23.41677564524290744, 35.51856778792605240, 6.000000000000000000 ) ) ;
#14160=VECTOR ( 'NONE', #18289, 1000.000000000000000 ) ;
#14163=ORIENTED_EDGE ( 'NONE', *, *, #18157, .T. ) ;
#14220=VERTEX_POINT ( 'NONE', #21672 ) ;
#14238=CARTESIAN_POINT ( 'NONE',  ( -6.000000000000000000, 28.00000000000000000, -6.000000000000000000 ) ) ;
#14292=AXIS2_PLACEMENT_3D ( 'NONE', #14831, #22226, #5638 ) ;
#14299=PLANE ( 'NONE',  #16841 ) ;
#14369=SHAPE_DEFINITION_REPRESENTATION ( #8047, #8755 ) ;
#14370=DIRECTION ( 'NONE',  ( 0.000000000000000000, -1.000000000000000000, 0.000000000000000000 ) ) ;
#14389=ORIENTED_EDGE ( 'NONE', *, *, #19768, .T. ) ;
#14406=DIRECTION ( 'NONE',  ( 0.000000000000000000, 1.000000000000000000, 0.000000000000000000 ) ) ;
#14422=VECTOR ( 'NONE', #13817, 1000.000000000000000 ) ;
#14457=PRESENTATION_STYLE_ASSIGNMENT (( #20037 ) ) ;
#14473=AXIS2_PLACEMENT_3D ( 'NONE', #18442, #2196, #11299 ) ;
#14474=VERTEX_POINT ( 'NONE', #4438 ) ;
#14518=AXIS2_PLACEMENT_3D ( 'NONE', #15611, #19011, #7879 ) ;
#14524=DIRECTION ( 'NONE',  ( 0.000000000000000000, -1.000000000000000000, 0.000000000000000000 ) ) ;
#14527=CARTESIAN_POINT ( 'NONE',  ( 2.649999999999999911, 26.50000000000000000, 0.000000000000000000 ) ) ;
#14553=VECTOR ( 'NONE', #15519, 1000.000000000000000 ) ;
#14661=DIRECTION ( 'NONE',  ( -0.4247135072049882942, 0.9053278062655749636, 0.000000000000000000 ) ) ;
#14749=DIRECTION ( 'NONE',  ( 0.000000000000000000, 1.000000000000000000, 0.000000000000000000 ) ) ;
#14752=ORIENTED_EDGE ( 'NONE', *, *, #22715, .T. ) ;
#14781=DIRECTION ( 'NONE',  ( 0.000000000000000000, 0.000000000000000000, -1.000000000000000000 ) ) ;
#14793=EDGE_LOOP ( 'NONE', ( #11182, #545 ) ) ;
#14831=CARTESIAN_POINT ( 'NONE',  ( 7.500000000000000000, 26.50000000000000000, -6.000000000000000000 ) ) ;
#14865=VERTEX_POINT ( 'NONE', #19242 ) ;
#14866=ADVANCED_FACE ( 'NONE', ( #21182 ), #2655, .F. ) ;
#14887=PLANE ( 'NONE',  #2801 ) ;
#14944=CARTESIAN_POINT ( 'NONE',  ( 61.60588651278290939, 37.01856778792605240, -6.000000000000000000 ) ) ;
#14966=VERTEX_POINT ( 'NONE', #13662 ) ;
#14978=PLANE ( 'NONE',  #6775 ) ;
#14998=CARTESIAN_POINT ( 'NONE',  ( 23.41677564524290744, 34.01856778792605240, -6.000000000000005329 ) ) ;
#15000=SHAPE_REPRESENTATION_RELATIONSHIP ( 'NONE' , 'NONE' ,  #8755, #23512 ) ;
#15007=ORIENTED_EDGE ( 'NONE', *, *, #5389, .T. ) ;
#15011=AXIS2_PLACEMENT_3D ( 'NONE', #10998, #7120, #1792 ) ;
#15022=ORIENTED_EDGE ( 'NONE', *, *, #5689, .T. ) ;
#15034=ADVANCED_FACE ( 'NONE', ( #789 ), #15439, .F. ) ;
#15064=CARTESIAN_POINT ( 'NONE',  ( -0.7783053373570000266, 26.50000000000000000, 5.000000000000000000 ) ) ;
#15080=CARTESIAN_POINT ( 'NONE',  ( 21.45754691133475944, 36.29044427405463580, -6.000000000000000000 ) ) ;
#15105=ORIENTED_EDGE ( 'NONE', *, *, #16296, .T. ) ;
#15115=DIRECTION ( 'NONE',  ( 0.000000000000000000, -1.000000000000000000, 0.000000000000000000 ) ) ;
#15118=EDGE_LOOP ( 'NONE', ( #6776, #13557, #1639, #1290 ) ) ;
#15136=VECTOR ( 'NONE', #12133, 1000.000000000000000 ) ;
#15147=AXIS2_PLACEMENT_3D ( 'NONE', #18539, #23515, #14661 ) ;
#15163=EDGE_CURVE ( 'NONE', #15717, #10339, #18722, .T. ) ;
#15211=LINE ( 'NONE', #7963, #3499 ) ;
#15226=CARTESIAN_POINT ( 'NONE',  ( 8.196152422706999729, 26.90192378864669820, 6.000000000000000000 ) ) ;
#15241=VERTEX_POINT ( 'NONE', #17883 ) ;
#15246=FACE_OUTER_BOUND ( 'NONE', #19709, .T. ) ;
#15249=LINE ( 'NONE', #4256, #6931 ) ;
#15258=ORIENTED_EDGE ( 'NONE', *, *, #3156, .F. ) ;
#15280=VERTEX_POINT ( 'NONE', #14238 ) ;
#15319=CARTESIAN_POINT ( 'NONE',  ( -6.046589298277226909, 26.49999999999999645, 1.190688249984996006 ) ) ;
#15323=VECTOR ( 'NONE', #11702, 1000.000000000000000 ) ;
#15339=EDGE_LOOP ( 'NONE', ( #22385, #5343, #9072, #17479 ) ) ;
#15347=AXIS2_PLACEMENT_3D ( 'NONE', #6342, #8289, #21252 ) ;
#15386=ORIENTED_EDGE ( 'NONE', *, *, #4462, .T. ) ;
#15412=AXIS2_PLACEMENT_3D ( 'NONE', #11054, #9119, #16492 ) ;
#15439=PLANE ( 'NONE',  #7649 ) ;
#15477=LINE ( 'NONE', #15226, #3145 ) ;
#15495=DIRECTION ( 'NONE',  ( 1.000000000000000000, 0.000000000000000000, 0.000000000000000000 ) ) ;
#15519=DIRECTION ( 'NONE',  ( 0.000000000000000000, 0.000000000000000000, 1.000000000000000000 ) ) ;
#15533=ADVANCED_FACE ( 'NONE', ( #13616 ), #22344, .T. ) ;
#15554=ORIENTED_EDGE ( 'NONE', *, *, #5142, .T. ) ;
#15561=CARTESIAN_POINT ( 'NONE',  ( -6.281924650935041932, 26.47351824524191954, 1.064721106944196416 ) ) ;
#15581=ORIENTED_EDGE ( 'NONE', *, *, #23747, .T. ) ;
#15585=EDGE_CURVE ( 'NONE', #18186, #9739, #11696, .T. ) ;
#15592=DIRECTION ( 'NONE',  ( 0.8660254037844288266, 0.5000000000000169864, 0.000000000000000000 ) ) ;
#15602=EDGE_CURVE ( 'NONE', #15754, #9702, #18956, .T. ) ;
#15611=CARTESIAN_POINT ( 'NONE',  ( 23.75352077758000036, 36.75000000000000000, -6.000000000000000000 ) ) ;
#15623=CARTESIAN_POINT ( 'NONE',  ( 66.60588651278291650, 37.01856778792605240, -1.000000000000000000 ) ) ;
#15624=ORIENTED_EDGE ( 'NONE', *, *, #3593, .T. ) ;
#15650=VERTEX_POINT ( 'NONE', #535 ) ;
#15655=ORIENTED_EDGE ( 'NONE', *, *, #22715, .F. ) ;
#15657=CARTESIAN_POINT ( 'NONE',  ( -3.657438266360000245, 84.95442836047000412, 3.657438266360000245 ) ) ;
#15665=PLANE ( 'NONE',  #12548 ) ;
#15709=AXIS2_PLACEMENT_3D ( 'NONE', #12222, #12463, #21304 ) ;
#15717=VERTEX_POINT ( 'NONE', #10118 ) ;
#15718=CARTESIAN_POINT ( 'NONE',  ( 22.66677564524290744, 35.31760589360604996, 6.000000000000000000 ) ) ;
#15733=AXIS2_PLACEMENT_3D ( 'NONE', #10758, #18258, #21889 ) ;
#15751=DIRECTION ( 'NONE',  ( 0.000000000000000000, 0.000000000000000000, 1.000000000000000000 ) ) ;
#15754=VERTEX_POINT ( 'NONE', #8552 ) ;
#15770=PLANE ( 'NONE',  #1047 ) ;
#15782=CIRCLE ( 'NONE', #13466, 2.673746900119611247 ) ;
#15787=FACE_OUTER_BOUND ( 'NONE', #23033, .T. ) ;
#15806=AXIS2_PLACEMENT_3D ( 'NONE', #21077, #20960, #4488 ) ;
#15838=DIRECTION ( 'NONE',  ( 0.4226182617406808451, 0.000000000000000000, -0.9063077870366587074 ) ) ;
#15887=ORIENTED_EDGE ( 'NONE', *, *, #3608, .F. ) ;
#15891=VERTEX_POINT ( 'NONE', #8623 ) ;
#15897=ORIENTED_EDGE ( 'NONE', *, *, #5144, .F. ) ;
#15902=CARTESIAN_POINT ( 'NONE',  ( -5.730762473771000565, 26.50000000000000000, 1.577381738259000077 ) ) ;
#15971=ADVANCED_FACE ( 'NONE', ( #17588 ), #983, .T. ) ;
#15972=DIRECTION ( 'NONE',  ( 0.000000000000000000, -1.000000000000000000, 0.000000000000000000 ) ) ;
#15979=CARTESIAN_POINT ( 'NONE',  ( 23.41677564524290744, 34.01856778792605240, -6.000000000000005329 ) ) ;
#15986=ORIENTED_EDGE ( 'NONE', *, *, #19133, .T. ) ;
#16002=ORIENTED_EDGE ( 'NONE', *, *, #13261, .F. ) ;
#16046=EDGE_LOOP ( 'NONE', ( #1621, #16109, #19313, #10092, #1126, #23249 ) ) ;
#16077=ORIENTED_EDGE ( 'NONE', *, *, #1737, .F. ) ;
#16096=ORIENTED_EDGE ( 'NONE', *, *, #16757, .F. ) ;
#16105=DIRECTION ( 'NONE',  ( 0.000000000000000000, 0.000000000000000000, 1.000000000000000000 ) ) ;
#16109=ORIENTED_EDGE ( 'NONE', *, *, #2740, .T. ) ;
#16129=ORIENTED_EDGE ( 'NONE', *, *, #16310, .T. ) ;
#16140=EDGE_CURVE ( 'NONE', #22330, #23444, #23349, .T. ) ;
#16152=EDGE_CURVE ( 'NONE', #11775, #9971, #10889, .T. ) ;
#16174=ORIENTED_EDGE ( 'NONE', *, *, #10159, .T. ) ;
#16194=VECTOR ( 'NONE', #13646, 1000.000000000000000 ) ;
#16204=ADVANCED_FACE ( 'NONE', ( #20097 ), #1571, .F. ) ;
#16212=LINE ( 'NONE', #15718, #8095 ) ;
#16230=ORIENTED_EDGE ( 'NONE', *, *, #3708, .F. ) ;
#16264=CARTESIAN_POINT ( 'NONE',  ( -6.000000000000000000, 26.50000000000000000, -6.000000000000000000 ) ) ;
#16269=CARTESIAN_POINT ( 'NONE',  ( -6.000000000000000000, 24.99999999999999645, -115.0195023120000002 ) ) ;
#16279=VERTEX_POINT ( 'NONE', #1674 ) ;
#16287=DIRECTION ( 'NONE',  ( 0.000000000000000000, 0.000000000000000000, 1.000000000000000000 ) ) ;
#16296=EDGE_CURVE ( 'NONE', #6372, #2681, #12817, .T. ) ;
#16297=ORIENTED_EDGE ( 'NONE', *, *, #6838, .F. ) ;
#16310=EDGE_CURVE ( 'NONE', #15754, #23789, #4985, .T. ) ;
#16311=AXIS2_PLACEMENT_3D ( 'NONE', #13939, #4748, #10191 ) ;
#16318=VECTOR ( 'NONE', #2658, 1000.000000000000000 ) ;
#16344=ADVANCED_FACE ( 'NONE', ( #4668 ), #12052, .T. ) ;
#16366=LINE ( 'NONE', #12745, #18873 ) ;
#16418=AXIS2_PLACEMENT_3D ( 'NONE', #10581, #14781, #7162 ) ;
#16427=CIRCLE ( 'NONE', #18009, 2.673746900119611247 ) ;
#16440=CARTESIAN_POINT ( 'NONE',  ( 44.70988823752291097, 36.26856778792605240, -6.000000000000000000 ) ) ;
#16472=EDGE_LOOP ( 'NONE', ( #11656, #16297, #3578, #20296 ) ) ;
#16482=AXIS2_PLACEMENT_3D ( 'NONE', #3204, #21728, #10346 ) ;
#16492=DIRECTION ( 'NONE',  ( 0.5000000000000169864, -0.8660254037844289376, 0.000000000000000000 ) ) ;
#16559=CIRCLE ( 'NONE', #20429, 1.500000000000001332 ) ;
#16570=MANIFOLD_SOLID_BREP ( 'Stock-MAS-673-1', #336 ) ;
#16591=VECTOR ( 'NONE', #7447, 1000.000000000000000 ) ;
#16695=CARTESIAN_POINT ( 'NONE',  ( 8.196152422706999729, 26.90192378864669820, 6.000000000000000000 ) ) ;
#16751=PRODUCT_DEFINITION_FORMATION_WITH_SPECIFIED_SOURCE ( 'ANY', '', #483, .NOT_KNOWN. ) ;
#16756=DIRECTION ( 'NONE',  ( 0.000000000000000000, 0.000000000000000000, 1.000000000000000000 ) ) ;
#16757=EDGE_CURVE ( 'NONE', #14966, #23789, #20680, .T. ) ;
#16797=CARTESIAN_POINT ( 'NONE',  ( 7.278495274186999708, 27.32666689084959799, 6.000000000000000000 ) ) ;
#16798=EDGE_LOOP ( 'NONE', ( #23904, #615, #4733, #4388 ) ) ;
#16826=EDGE_LOOP ( 'NONE', ( #2660, #13703, #15581, #15022 ) ) ;
#16835=DIRECTION ( 'NONE',  ( -1.000000000000000000, 0.000000000000000000, 0.000000000000000000 ) ) ;
#16841=AXIS2_PLACEMENT_3D ( 'NONE', #12601, #8968, #1093 ) ;
#16870=ORIENTED_EDGE ( 'NONE', *, *, #16310, .F. ) ;
#16879=ORIENTED_EDGE ( 'NONE', *, *, #16140, .F. ) ;
#16888=DIRECTION ( 'NONE',  ( 0.9063077870366408328, 0.000000000000000000, -0.4226182617407188702 ) ) ;
#16901=VECTOR ( 'NONE', #19493, 1000.000000000000000 ) ;
#16911=AXIS2_PLACEMENT_3D ( 'NONE', #6735, #3126, #8568 ) ;
#16930=FACE_OUTER_BOUND ( 'NONE', #9112, .T. ) ;
#16952=ADVANCED_FACE ( 'NONE', ( #10517 ), #21405, .T. ) ;
#16998=CARTESIAN_POINT ( 'NONE',  ( -7.500000000000000000, 24.99999999999999645, -6.000000000000000000 ) ) ;
#17007=DIRECTION ( 'NONE',  ( 0.8660254037844288266, 0.5000000000000169864, 0.000000000000000000 ) ) ;
#17009=DIRECTION ( 'NONE',  ( 1.000000000000000000, 0.000000000000000000, 0.000000000000000000 ) ) ;
#17036=VERTEX_POINT ( 'NONE', #10867 ) ;
#17054=ORIENTED_EDGE ( 'NONE', *, *, #6460, .F. ) ;
#17058=CARTESIAN_POINT ( 'NONE',  ( 6.696152422707000618, 29.50000000000000000, -6.000000000000000000 ) ) ;
#17065=EDGE_CURVE ( 'NONE', #19197, #5360, #18361, .T. ) ;
#17071=CARTESIAN_POINT ( 'NONE',  ( -6.000000000000000000, 26.50000000000000000, -6.000000000000000000 ) ) ;
#17073=EDGE_CURVE ( 'NONE', #23198, #18177, #18020, .T. ) ;
#17076=EDGE_CURVE ( 'NONE', #15891, #9532, #9281, .T. ) ;
#17086=AXIS2_PLACEMENT_3D ( 'NONE', #15657, #773, #18947 ) ;
#17120=ADVANCED_FACE ( 'NONE', ( #9393 ), #9511, .F. ) ;
#17139=DIRECTION ( 'NONE',  ( 1.000000000000000000, 0.000000000000000000, 0.000000000000000000 ) ) ;
#17142=DIRECTION ( 'NONE',  ( 0.000000000000000000, 0.000000000000000000, -1.000000000000000000 ) ) ;
#17160=DIRECTION ( 'NONE',  ( 0.000000000000000000, -1.000000000000000000, 0.000000000000000000 ) ) ;
#17186=CARTESIAN_POINT ( 'NONE',  ( 8.196152422706999729, 26.90192378864669820, 6.000000000000000000 ) ) ;
#17206=DIRECTION ( 'NONE',  ( 0.000000000000000000, 0.000000000000000000, -1.000000000000000000 ) ) ;
#17257=EDGE_CURVE ( 'NONE', #13296, #11734, #8126, .T. ) ;
#17288=LINE ( 'NONE', #11846, #18931 ) ;
#17289=ORIENTED_EDGE ( 'NONE', *, *, #20077, .T. ) ;
#17294=DIRECTION ( 'NONE',  ( 0.000000000000000000, 1.000000000000000000, 0.000000000000000000 ) ) ;
#17319=CARTESIAN_POINT ( 'NONE',  ( -9.000000000000000000, 24.99999999999999645, -6.000000000000000000 ) ) ;
#17322=VERTEX_POINT ( 'NONE', #6175 ) ;
#17397=FACE_OUTER_BOUND ( 'NONE', #12293, .T. ) ;
#17431=DIRECTION ( 'NONE',  ( 0.000000000000000000, 0.000000000000000000, -1.000000000000000000 ) ) ;
#17455=ORIENTED_EDGE ( 'NONE', *, *, #22450, .F. ) ;
#17464=ORIENTED_EDGE ( 'NONE', *, *, #6460, .T. ) ;
#17479=ORIENTED_EDGE ( 'NONE', *, *, #13548, .T. ) ;
#17492=DIRECTION ( 'NONE',  ( 0.000000000000000000, 0.000000000000000000, -1.000000000000000000 ) ) ;
#17557=AXIS2_PLACEMENT_3D ( 'NONE', #23320, #4696, #14370 ) ;
#17564=ORIENTED_EDGE ( 'NONE', *, *, #4955, .F. ) ;
#17568=EDGE_CURVE ( 'NONE', #23444, #10297, #10827, .T. ) ;
#17572=PLANE ( 'NONE',  #14518 ) ;
#17588=FACE_OUTER_BOUND ( 'NONE', #21287, .T. ) ;
#17619=ORIENTED_EDGE ( 'NONE', *, *, #17065, .T. ) ;
#17643=CARTESIAN_POINT ( 'NONE',  ( 30.87226923053214378, 27.01856778792605240, -2.673746900119611247 ) ) ;
#17672=AXIS2_PLACEMENT_3D ( 'NONE', #21704, #10802, #16105 ) ;
#17700=DIRECTION ( 'NONE',  ( 0.000000000000000000, -1.000000000000000000, 0.000000000000000000 ) ) ;
#17710=ADVANCED_FACE ( 'NONE', ( #5185 ), #3707, .T. ) ;
#17726=EDGE_LOOP ( 'NONE', ( #10794, #1824, #1971, #15887 ) ) ;
#17782=CARTESIAN_POINT ( 'NONE',  ( 0.3480762113532999691, 27.25000000000000000, -6.000000000000000000 ) ) ;
#17817=LINE ( 'NONE', #5214, #5984 ) ;
#17855=EDGE_LOOP ( 'NONE', ( #16879, #12590, #11450, #23127 ) ) ;
#17883=CARTESIAN_POINT ( 'NONE',  ( 60.61494135913342518, 35.51856778792605240, -2.673746900119611247 ) ) ;
#17892=LINE ( 'NONE', #1042, #932 ) ;
#17937=DIRECTION ( 'NONE',  ( 1.000000000000000000, 0.000000000000000000, 0.000000000000000000 ) ) ;
#17953=APPLICATION_CONTEXT ( 'automotive_design' ) ;
#17956=EDGE_CURVE ( 'NONE', #10339, #9862, #10186, .T. ) ;
#17958=DIRECTION ( 'NONE',  ( -0.4226182617406808451, 0.000000000000000000, 0.9063077870366587074 ) ) ;
#17976=LINE ( 'NONE', #2958, #19699 ) ;
#17992=VECTOR ( 'NONE', #18188, 1000.000000000000000 ) ;
#18009=AXIS2_PLACEMENT_3D ( 'NONE', #12965, #3891, #12852 ) ;
#18015=LINE ( 'NONE', #8815, #11684 ) ;
#18020=LINE ( 'NONE', #9043, #16591 ) ;
#18147=VECTOR ( 'NONE', #18438, 1000.000000000000000 ) ;
#18157=EDGE_CURVE ( 'NONE', #15650, #6003, #19874, .T. ) ;
#18158=AXIS2_PLACEMENT_3D ( 'NONE', #22695, #7697, #16888 ) ;
#18160=VERTEX_POINT ( 'NONE', #21450 ) ;
#18168=CARTESIAN_POINT ( 'NONE',  ( -9.000000000000000000, 19.50000000000000000, -6.000000000000000000 ) ) ;
#18177=VERTEX_POINT ( 'NONE', #5108 ) ;
#18186=VERTEX_POINT ( 'NONE', #10795 ) ;
#18188=DIRECTION ( 'NONE',  ( 1.000000000000000000, 0.000000000000000000, 0.000000000000000000 ) ) ;
#18217=DIRECTION ( 'NONE',  ( 0.000000000000000000, 0.000000000000000000, 1.000000000000000000 ) ) ;
#18240=VERTEX_POINT ( 'NONE', #3290 ) ;
#18258=DIRECTION ( 'NONE',  ( 0.000000000000000000, 1.000000000000000000, 0.000000000000000000 ) ) ;
#18263=AXIS2_PLACEMENT_3D ( 'NONE', #12014, #17206, #21084 ) ;
#18279=LINE ( 'NONE', #18386, #729 ) ;
#18289=DIRECTION ( 'NONE',  ( 0.9063077870366585964, 0.000000000000000000, 0.4226182617406808451 ) ) ;
#18293=EDGE_LOOP ( 'NONE', ( #21219, #2243, #18839, #14752 ) ) ;
#18306=FACE_OUTER_BOUND ( 'NONE', #6, .T. ) ;
#18361=LINE ( 'NONE', #23583, #13493 ) ;
#18386=CARTESIAN_POINT ( 'NONE',  ( 7.446152422707000618, 28.20096189432300093, 6.000000000000000000 ) ) ;
#18416=CARTESIAN_POINT ( 'NONE',  ( -4.080056528100000079, 28.00000000000000000, 4.563746053395999702 ) ) ;
#18438=DIRECTION ( 'NONE',  ( 0.000000000000000000, 0.000000000000000000, 1.000000000000000000 ) ) ;
#18442=CARTESIAN_POINT ( 'NONE',  ( 0.3480762113532999691, 27.25000000000000000, 6.000000000000000000 ) ) ;
#18452=CARTESIAN_POINT ( 'NONE',  ( 60.61494135913342518, 37.01856778792605240, 2.673746900119611247 ) ) ;
#18525=ORIENTED_EDGE ( 'NONE', *, *, #18603, .T. ) ;
#18534=( NAMED_UNIT ( * ) SI_UNIT ( $, .STERADIAN. ) SOLID_ANGLE_UNIT ( ) );
#18539=CARTESIAN_POINT ( 'NONE',  ( -6.000000000000000000, 24.99999999999999645, 1.000000000000000000 ) ) ;
#18554=ORIENTED_EDGE ( 'NONE', *, *, #10737, .T. ) ;
#18568=ORIENTED_EDGE ( 'NONE', *, *, #22088, .F. ) ;
#18570=FACE_OUTER_BOUND ( 'NONE', #17855, .T. ) ;
#18595=LINE ( 'NONE', #3587, #7909 ) ;
#18603=EDGE_CURVE ( 'NONE', #14220, #14865, #11667, .T. ) ;
#18615=CARTESIAN_POINT ( 'NONE',  ( 22.66677564524435340, 35.31760589360354885, -6.000000000000000000 ) ) ;
#18674=DIRECTION ( 'NONE',  ( 0.000000000000000000, -1.000000000000000000, 0.000000000000000000 ) ) ;
#18705=LINE ( 'NONE', #9980, #21022 ) ;
#18707=ORIENTED_EDGE ( 'NONE', *, *, #23593, .F. ) ;
#18714=CARTESIAN_POINT ( 'NONE',  ( 23.41677564524290744, 35.51856778792605240, -6.000000000000000000 ) ) ;
#18719=EDGE_CURVE ( 'NONE', #14865, #611, #12509, .T. ) ;
#18722=LINE ( 'NONE', #6115, #15323 ) ;
#18725=AXIS2_PLACEMENT_3D ( 'NONE', #10625, #16756, #5514 ) ;
#18746=DIRECTION ( 'NONE',  ( 0.000000000000000000, 0.000000000000000000, -1.000000000000000000 ) ) ;
#18747=VECTOR ( 'NONE', #470, 1000.000000000000000 ) ;
#18777=ORIENTED_EDGE ( 'NONE', *, *, #4655, .F. ) ;
#18814=ORIENTED_EDGE ( 'NONE', *, *, #18719, .T. ) ;
#18823=ADVANCED_FACE ( 'NONE', ( #19538 ), #23269, .F. ) ;
#18839=ORIENTED_EDGE ( 'NONE', *, *, #14134, .F. ) ;
#18847=CARTESIAN_POINT ( 'NONE',  ( -6.000000000000000000, 26.50000000000000000, 1.229194263906000062 ) ) ;
#18849=EDGE_CURVE ( 'NONE', #9971, #11154, #12595, .T. ) ;
#18873=VECTOR ( 'NONE', #7159, 1000.000000000000000 ) ;
#18883=EDGE_CURVE ( 'NONE', #7660, #17322, #16427, .T. ) ;
#18931=VECTOR ( 'NONE', #560, 1000.000000000000000 ) ;
#18947=DIRECTION ( 'NONE',  ( -0.4226182617406811226, 0.000000000000000000, 0.9063077870366585964 ) ) ;
#18954=CARTESIAN_POINT ( 'NONE',  ( -6.000000000000000000, 26.50000000000000000, 1.229194263906000062 ) ) ;
#18956=LINE ( 'NONE', #9753, #8401 ) ;
#18973=CARTESIAN_POINT ( 'NONE',  ( -7.500000000000000000, 19.50000000000000000, -6.000000000000000000 ) ) ;
#18977=DIRECTION ( 'NONE',  ( 0.000000000000000000, -1.000000000000000000, 0.000000000000000000 ) ) ;
#18990=VERTEX_POINT ( 'NONE', #20361 ) ;
#19008=DIRECTION ( 'NONE',  ( 0.000000000000000000, 1.000000000000000000, 0.000000000000000000 ) ) ;
#19011=DIRECTION ( 'NONE',  ( 0.000000000000000000, 0.000000000000000000, -1.000000000000000000 ) ) ;
#19072=DIRECTION ( 'NONE',  ( 0.5000000000000172085, -0.8660254037844288266, 0.000000000000000000 ) ) ;
#19100=CIRCLE ( 'NONE', #2473, 2.999999999999999112 ) ;
#19105=EDGE_CURVE ( 'NONE', #21343, #15280, #21069, .T. ) ;
#19133=EDGE_CURVE ( 'NONE', #23444, #14865, #17817, .T. ) ;
#19137=ORIENTED_EDGE ( 'NONE', *, *, #11710, .T. ) ;
#19147=EDGE_LOOP ( 'NONE', ( #7105, #22532, #640, #15258, #7783, #11201 ) ) ;
#19194=DIRECTION ( 'NONE',  ( 0.000000000000000000, 1.000000000000000000, 0.000000000000000000 ) ) ;
#19197=VERTEX_POINT ( 'NONE', #6898 ) ;
#19204=CARTESIAN_POINT ( 'NONE',  ( 23.41677564524290744, 34.01856778792605240, -115.0195023120000002 ) ) ;
#19242=CARTESIAN_POINT ( 'NONE',  ( -7.500000000000000000, 22.00000000000000000, -1.000000000000000000 ) ) ;
#19247=CARTESIAN_POINT ( 'NONE',  ( -9.000000000000000000, 19.50000000000000000, -5.000000000000000000 ) ) ;
#19313=ORIENTED_EDGE ( 'NONE', *, *, #5257, .T. ) ;
#19346=ORIENTED_EDGE ( 'NONE', *, *, #15585, .T. ) ;
#19348=ADVANCED_FACE ( 'NONE', ( #3625 ), #5325, .T. ) ;
#19413=ADVANCED_FACE ( 'NONE', ( #21912, #3976 ), #14978, .T. ) ;
#19466=EDGE_LOOP ( 'NONE', ( #10467, #15554, #1253, #4341, #8565, #11834, #16129, #18777, #22823 ) ) ;
#19467=LINE ( 'NONE', #18973, #4159 ) ;
#19473=EDGE_CURVE ( 'NONE', #10339, #14083, #19961, .T. ) ;
#19493=DIRECTION ( 'NONE',  ( 1.000000000000000000, 0.000000000000000000, 0.000000000000000000 ) ) ;
#19500=VERTEX_POINT ( 'NONE', #11844 ) ;
#19501=DIRECTION ( 'NONE',  ( -0.5000000000000169864, 0.8660254037844288266, 0.000000000000000000 ) ) ;
#19538=FACE_OUTER_BOUND ( 'NONE', #20357, .T. ) ;
#19546=CARTESIAN_POINT ( 'NONE',  ( -7.590990257669999686, 26.59099025766972701, -6.000000000000000000 ) ) ;
#19581=VECTOR ( 'NONE', #20025, 1000.000000000000000 ) ;
#19598=CIRCLE ( 'NONE', #19993, 1.000000000000000666 ) ;
#19622=ORIENTED_EDGE ( 'NONE', *, *, #11891, .F. ) ;
#19634=CIRCLE ( 'NONE', #15347, 2.999999999999999112 ) ;
#19663=ORIENTED_EDGE ( 'NONE', *, *, #3608, .T. ) ;
#19668=EDGE_LOOP ( 'NONE', ( #21112, #1470, #16077, #15897 ) ) ;
#19673=CARTESIAN_POINT ( 'NONE',  ( -7.500000000000000000, 18.50000000000000000, -5.000000000000000000 ) ) ;
#19690=CIRCLE ( 'NONE', #12343, 5.000000000000004441 ) ;
#19699=VECTOR ( 'NONE', #21485, 1000.000000000000000 ) ;
#19701=CYLINDRICAL_SURFACE ( 'NONE', #5279, 3.000000000000000000 ) ;
#19709=EDGE_LOOP ( 'NONE', ( #4532, #3138, #6053, #14163 ) ) ;
#19747=CARTESIAN_POINT ( 'NONE',  ( 6.696152422707000618, 26.50000000000000000, 6.000000000000000000 ) ) ;
#19759=CARTESIAN_POINT ( 'NONE',  ( -5.730762473771000565, 28.00000000000000000, 1.577381738259000077 ) ) ;
#19768=EDGE_CURVE ( 'NONE', #11438, #13125, #21324, .T. ) ;
#19786=ADVANCED_FACE ( 'NONE', ( #15246 ), #722, .F. ) ;
#19826=PLANE ( 'NONE',  #18725 ) ;
#19830=CARTESIAN_POINT ( 'NONE',  ( -4.080056528100000079, 26.50000000000000000, 4.563746053395999702 ) ) ;
#19854=DIRECTION ( 'NONE',  ( 0.000000000000000000, -1.000000000000000000, 0.000000000000000000 ) ) ;
#19874=LINE ( 'NONE', #12605, #17992 ) ;
#19876=LINE ( 'NONE', #11020, #4991 ) ;
#19890=ORIENTED_EDGE ( 'NONE', *, *, #17073, .T. ) ;
#19897=EDGE_CURVE ( 'NONE', #14474, #10297, #11642, .T. ) ;
#19906=ADVANCED_FACE ( 'NONE', ( #22882 ), #17572, .T. ) ;
#19908=DIRECTION ( 'NONE',  ( -0.9063077870366409439, 0.000000000000000000, 0.4226182617407191477 ) ) ;
#19920=FILL_AREA_STYLE ('',( #7073 ) ) ;
#19951=EDGE_CURVE ( 'NONE', #18160, #11418, #6782, .T. ) ;
#19961=CIRCLE ( 'NONE', #20327, 5.000000000000000000 ) ;
#19993=AXIS2_PLACEMENT_3D ( 'NONE', #1136, #12522, #19908 ) ;
#19994=DIRECTION ( 'NONE',  ( 0.000000000000000000, 0.000000000000000000, -1.000000000000000000 ) ) ;
#20006=ORIENTED_EDGE ( 'NONE', *, *, #1276, .T. ) ;
#20011=CARTESIAN_POINT ( 'NONE',  ( 0.000000000000000000, 28.00000000000000000, 0.000000000000000000 ) ) ;
#20018=ADVANCED_FACE ( 'NONE', ( #6906 ), #14299, .F. ) ;
#20025=DIRECTION ( 'NONE',  ( 0.000000000000000000, 0.000000000000000000, 1.000000000000000000 ) ) ;
#20037=SURFACE_STYLE_USAGE ( .BOTH. , #5037 ) ;
#20072=DIRECTION ( 'NONE',  ( 0.000000000000000000, 0.000000000000000000, 1.000000000000000000 ) ) ;
#20077=EDGE_CURVE ( 'NONE', #23198, #14966, #22256, .T. ) ;
#20079=ORIENTED_EDGE ( 'NONE', *, *, #7257, .T. ) ;
#20097=FACE_OUTER_BOUND ( 'NONE', #17726, .T. ) ;
#20100=UNCERTAINTY_MEASURE_WITH_UNIT (LENGTH_MEASURE( 1.000000000000000082E-05 ), #6831, 'distance_accuracy_value', 'NONE');
#20102=PLANE ( 'NONE',  #21641 ) ;
#20157=ORIENTED_EDGE ( 'NONE', *, *, #23593, .T. ) ;
#20165=ADVANCED_FACE ( 'NONE', ( #1689, #329 ), #2157, .T. ) ;
#20180=EDGE_CURVE ( 'NONE', #5053, #19500, #7734, .T. ) ;
#20181=ORIENTED_EDGE ( 'NONE', *, *, #4322, .F. ) ;
#20256=ORIENTED_EDGE ( 'NONE', *, *, #11562, .F. ) ;
#20278=AXIS2_PLACEMENT_3D ( 'NONE', #19247, #10053, #8118 ) ;
#20296=ORIENTED_EDGE ( 'NONE', *, *, #20786, .F. ) ;
#20323=CARTESIAN_POINT ( 'NONE',  ( 21.45754691133435799, 36.29044427405532502, 6.000000000000005329 ) ) ;
#20325=LINE ( 'NONE', #1576, #12040 ) ;
#20327=AXIS2_PLACEMENT_3D ( 'NONE', #10898, #14749, #3861 ) ;
#20333=ORIENTED_EDGE ( 'NONE', *, *, #18883, .T. ) ;
#20352=ADVANCED_FACE ( 'NONE', ( #5166 ), #19701, .T. ) ;
#20357=EDGE_LOOP ( 'NONE', ( #20157, #19663, #4018, #14059 ) ) ;
#20361=CARTESIAN_POINT ( 'NONE',  ( 60.61494135913342518, 37.01856778792605240, -2.673746900119611247 ) ) ;
#20429=AXIS2_PLACEMENT_3D ( 'NONE', #9084, #19994, #23624 ) ;
#20438=DIRECTION ( 'NONE',  ( 0.000000000000000000, 1.000000000000000000, 0.000000000000000000 ) ) ;
#20439=CIRCLE ( 'NONE', #8865, 1.000000000000000666 ) ;
#20450=CIRCLE ( 'NONE', #8076, 2.649999999999999911 ) ;
#20483=VECTOR ( 'NONE', #6209, 1000.000000000000000 ) ;
#20488=CARTESIAN_POINT ( 'NONE',  ( 0.000000000000000000, 26.50000000000000000, 0.000000000000000000 ) ) ;
#20567=DIRECTION ( 'NONE',  ( 0.000000000000000000, -1.000000000000000000, 0.000000000000000000 ) ) ;
#20586=CYLINDRICAL_SURFACE ( 'NONE', #9384, 5.000000000000004441 ) ;
#20617=CARTESIAN_POINT ( 'NONE',  ( -0.7783053373570000266, 28.00000000000000000, 6.000000000000000000 ) ) ;
#20630=ORIENTED_EDGE ( 'NONE', *, *, #13519, .T. ) ;
#20651=CARTESIAN_POINT ( 'NONE',  ( 23.41677564524290744, 37.01856778792605240, -6.000000000000000000 ) ) ;
#20666=VECTOR ( 'NONE', #11565, 1000.000000000000000 ) ;
#20668=ORIENTED_EDGE ( 'NONE', *, *, #20798, .T. ) ;
#20680=LINE ( 'NONE', #22370, #13102 ) ;
#20689=AXIS2_PLACEMENT_3D ( 'NONE', #2943, #23644, #12272 ) ;
#20722=CARTESIAN_POINT ( 'NONE',  ( 66.60588651278291650, 37.01856778792605240, -1.000000000000000000 ) ) ;
#20738=ORIENTED_EDGE ( 'NONE', *, *, #14134, .T. ) ;
#20755=EDGE_CURVE ( 'NONE', #6003, #10297, #12283, .T. ) ;
#20759=ORIENTED_EDGE ( 'NONE', *, *, #17956, .F. ) ;
#20761=EDGE_CURVE ( 'NONE', #15280, #11438, #12232, .T. ) ;
#20762=DIRECTION ( 'NONE',  ( 0.6370702608075069495, 0.000000000000000000, -0.7708057360935083313 ) ) ;
#20786=EDGE_CURVE ( 'NONE', #18240, #13009, #1009, .T. ) ;
#20788=DIRECTION ( 'NONE',  ( 0.000000000000000000, -1.000000000000000000, 0.000000000000000000 ) ) ;
#20798=EDGE_CURVE ( 'NONE', #11418, #23198, #19598, .T. ) ;
#20808=VERTEX_POINT ( 'NONE', #2190 ) ;
#20829=ORIENTED_EDGE ( 'NONE', *, *, #1977, .T. ) ;
#20841=DIRECTION ( 'NONE',  ( 1.000000000000000000, 0.000000000000000000, 0.000000000000000000 ) ) ;
#20861=CIRCLE ( 'NONE', #1529, 3.000000000000001332 ) ;
#20872=DIRECTION ( 'NONE',  ( 1.000000000000000000, 0.000000000000000000, 0.000000000000000000 ) ) ;
#20898=DIRECTION ( 'NONE',  ( 0.000000000000000000, 1.000000000000000000, 0.000000000000000000 ) ) ;
#20905=CARTESIAN_POINT ( 'NONE',  ( -4.563746053395999702, 28.00000000000000000, 4.080056528100000079 ) ) ;
#20907=DIRECTION ( 'NONE',  ( 0.000000000000000000, -1.000000000000000000, 0.000000000000000000 ) ) ;
#20910=CARTESIAN_POINT ( 'NONE',  ( -6.253205914068437288, 26.47872451769842783, 1.076069669024710906 ) ) ;
#20922=DIRECTION ( 'NONE',  ( 0.000000000000000000, 0.000000000000000000, -1.000000000000000000 ) ) ;
#20937=ORIENTED_EDGE ( 'NONE', *, *, #9850, .F. ) ;
#20960=DIRECTION ( 'NONE',  ( 0.000000000000000000, -1.000000000000000000, 0.000000000000000000 ) ) ;
#20971=DIRECTION ( 'NONE',  ( 1.000000000000000000, 0.000000000000000000, 0.000000000000000000 ) ) ;
#21006=DIRECTION ( 'NONE',  ( 0.000000000000000000, -1.000000000000000000, 0.000000000000000000 ) ) ;
#21022=VECTOR ( 'NONE', #17007, 1000.000000000000114 ) ;
#21024=EDGE_LOOP ( 'NONE', ( #4716, #22897, #6729, #20937 ) ) ;
#21069=LINE ( 'NONE', #17071, #18747 ) ;
#21072=CYLINDRICAL_SURFACE ( 'NONE', #23902, 2.649999999999999911 ) ;
#21077=CARTESIAN_POINT ( 'NONE',  ( 61.60588651278290939, 74.97299614839606363, -1.000000000000000000 ) ) ;
#21084=DIRECTION ( 'NONE',  ( -0.5000000000000167644, 0.8660254037844290487, 0.000000000000000000 ) ) ;
#21112=ORIENTED_EDGE ( 'NONE', *, *, #19105, .T. ) ;
#21117=LINE ( 'NONE', #2465, #11877 ) ;
#21121=ORIENTED_EDGE ( 'NONE', *, *, #5389, .F. ) ;
#21124=LINE ( 'NONE', #2591, #10603 ) ;
#21138=EDGE_LOOP ( 'NONE', ( #5110, #5576, #13977, #11030 ) ) ;
#21156=EDGE_LOOP ( 'NONE', ( #12318, #22550, #9431, #3968, #9781 ) ) ;
#21182=FACE_OUTER_BOUND ( 'NONE', #7174, .T. ) ;
#21196=DIRECTION ( 'NONE',  ( 1.000000000000000000, 0.000000000000000000, 0.000000000000000000 ) ) ;
#21203=ORIENTED_EDGE ( 'NONE', *, *, #8544, .T. ) ;
#21219=ORIENTED_EDGE ( 'NONE', *, *, #15602, .T. ) ;
#21245=AXIS2_PLACEMENT_3D ( 'NONE', #8610, #15972, #17937 ) ;
#21247=ADVANCED_FACE ( 'NONE', ( #7002, #1318 ), #21422, .F. ) ;
#21252=DIRECTION ( 'NONE',  ( -1.000000000000000000, 0.000000000000000000, 0.000000000000000000 ) ) ;
#21278=DIRECTION ( 'NONE',  ( -1.000000000000000000, 0.000000000000000000, 0.000000000000000000 ) ) ;
#21283=AXIS2_PLACEMENT_3D ( 'NONE', #16797, #6017, #18977 ) ;
#21287=EDGE_LOOP ( 'NONE', ( #5911, #10943, #14097, #12647 ) ) ;
#21288=DIRECTION ( 'NONE',  ( 0.000000000000000000, 1.000000000000000000, 0.000000000000000000 ) ) ;
#21302=CARTESIAN_POINT ( 'NONE',  ( -6.000000000000000000, 28.00000000000000000, 1.229194263906999929 ) ) ;
#21304=DIRECTION ( 'NONE',  ( 0.000000000000000000, 0.000000000000000000, -1.000000000000000000 ) ) ;
#21306=CARTESIAN_POINT ( 'NONE',  ( -0.7783053373570000266, 28.00000000000000000, 6.000000000000000000 ) ) ;
#21318=CIRCLE ( 'NONE', #25, 1.500000000000000222 ) ;
#21324=LINE ( 'NONE', #17319, #1764 ) ;
#21343=VERTEX_POINT ( 'NONE', #21783 ) ;
#21401=DIRECTION ( 'NONE',  ( 0.9063077870366585964, 0.000000000000000000, 0.4226182617406808451 ) ) ;
#21405=PLANE ( 'NONE',  #11573 ) ;
#21415=AXIS2_PLACEMENT_3D ( 'NONE', #16269, #10946, #12529 ) ;
#21422=PLANE ( 'NONE',  #15709 ) ;
#21430=CARTESIAN_POINT ( 'NONE',  ( -2.704962792832999785, 27.25000000000000000, 5.204962792833000229 ) ) ;
#21450=CARTESIAN_POINT ( 'NONE',  ( -5.730762473771000565, 28.00000000000000000, 1.577381738259000077 ) ) ;
#21464=DIRECTION ( 'NONE',  ( 0.000000000000000000, -1.000000000000000000, 0.000000000000000000 ) ) ;
#21485=DIRECTION ( 'NONE',  ( 0.000000000000000000, 1.000000000000000000, 0.000000000000000000 ) ) ;
#21514=VECTOR ( 'NONE', #22495, 1000.000000000000000 ) ;
#21569=EDGE_CURVE ( 'NONE', #23889, #23570, #21117, .T. ) ;
#21586=CARTESIAN_POINT ( 'NONE',  ( 66.60588651278291650, 35.51856778792605240, 1.000000000000000000 ) ) ;
#21597=CARTESIAN_POINT ( 'NONE',  ( -7.500000000000000000, 22.00000000000000000, -1.000000000000000000 ) ) ;
#21638=CYLINDRICAL_SURFACE ( 'NONE', #10816, 3.000000000000002665 ) ;
#21641=AXIS2_PLACEMENT_3D ( 'NONE', #16440, #3512, #10893 ) ;
#21648=EDGE_CURVE ( 'NONE', #22330, #611, #881, .T. ) ;
#21672=CARTESIAN_POINT ( 'NONE',  ( -7.500000000000000000, 22.00000000000000000, 1.000000000000000000 ) ) ;
#21704=CARTESIAN_POINT ( 'NONE',  ( 30.87226923053214378, 27.01856778792605240, 0.000000000000000000 ) ) ;
#21706=CARTESIAN_POINT ( 'NONE',  ( 23.41677564524290744, 35.51856778792605240, 6.000000000000000000 ) ) ;
#21723=DIRECTION ( 'NONE',  ( 0.000000000000000000, -1.000000000000000000, 0.000000000000000000 ) ) ;
#21728=DIRECTION ( 'NONE',  ( 0.000000000000000000, -1.000000000000000000, 0.000000000000000000 ) ) ;
#21737=EDGE_LOOP ( 'NONE', ( #15986, #18814, #4758, #1756 ) ) ;
#21783=CARTESIAN_POINT ( 'NONE',  ( -6.000000000000000000, 26.50000000000000000, -6.000000000000000000 ) ) ;
#21812=DIRECTION ( 'NONE',  ( 0.000000000000000000, 0.000000000000000000, -1.000000000000000000 ) ) ;
#21834=CARTESIAN_POINT ( 'NONE',  ( -7.500000000000000000, 19.50000000000000000, -5.000000000000000000 ) ) ;
#21835=ADVANCED_FACE ( 'NONE', ( #1352 ), #8743, .F. ) ;
#21873=ORIENTED_EDGE ( 'NONE', *, *, #16152, .F. ) ;
#21889=DIRECTION ( 'NONE',  ( 1.000000000000000000, 0.000000000000000000, 0.000000000000000000 ) ) ;
#21912=FACE_BOUND ( 'NONE', #7374, .T. ) ;
#21951=VECTOR ( 'NONE', #7143, 1000.000000000000000 ) ;
#21967=CARTESIAN_POINT ( 'NONE',  ( 22.83443279375291368, 36.19190089707605296, 6.000000000000000000 ) ) ;
#21990=ORIENTED_EDGE ( 'NONE', *, *, #20755, .F. ) ;
#21997=VECTOR ( 'NONE', #8335, 1000.000000000000000 ) ;
#22010=AXIS2_PLACEMENT_3D ( 'NONE', #9249, #2209, #22989 ) ;
#22027=CIRCLE ( 'NONE', #11587, 2.673746900119611247 ) ;
#22052=( LENGTH_UNIT ( ) NAMED_UNIT ( * ) SI_UNIT ( .MILLI., .METRE. ) );
#22053=ORIENTED_EDGE ( 'NONE', *, *, #13234, .T. ) ;
#22088=EDGE_CURVE ( 'NONE', #11775, #3633, #9555, .T. ) ;
#22105=PRODUCT_CONTEXT ( 'NONE', #17953, 'mechanical' ) ;
#22182=ORIENTED_EDGE ( 'NONE', *, *, #15163, .T. ) ;
#22187=ADVANCED_FACE ( 'NONE', ( #7058 ), #15770, .F. ) ;
#22215=ORIENTED_EDGE ( 'NONE', *, *, #12790, .T. ) ;
#22218=VECTOR ( 'NONE', #7906, 1000.000000000000000 ) ;
#22226=DIRECTION ( 'NONE',  ( 0.5000000000000169864, -0.8660254037844288266, 0.000000000000000000 ) ) ;
#22241=LINE ( 'NONE', #9419, #6082 ) ;
#22256=LINE ( 'NONE', #7250, #14160 ) ;
#22275=FACE_OUTER_BOUND ( 'NONE', #9676, .T. ) ;
#22276=CARTESIAN_POINT ( 'NONE',  ( 6.750000000000000000, 27.79903810567699907, -6.000000000000000000 ) ) ;
#22330=VERTEX_POINT ( 'NONE', #1373 ) ;
#22333=AXIS2_PLACEMENT_3D ( 'NONE', #1013, #17492, #23542 ) ;
#22344=PLANE ( 'NONE',  #7603 ) ;
#22370=CARTESIAN_POINT ( 'NONE',  ( -1.200923599098000061, 28.00000000000000000, 5.906307787036999990 ) ) ;
#22379=EDGE_LOOP ( 'NONE', ( #8014, #19622, #512, #18707 ) ) ;
#22385=ORIENTED_EDGE ( 'NONE', *, *, #12227, .T. ) ;
#22418=ORIENTED_EDGE ( 'NONE', *, *, #22450, .T. ) ;
#22437=DIRECTION ( 'NONE',  ( 0.000000000000000000, 0.000000000000000000, 1.000000000000000000 ) ) ;
#22450=EDGE_CURVE ( 'NONE', #9818, #4666, #19634, .T. ) ;
#22493=ORIENTED_EDGE ( 'NONE', *, *, #10737, .F. ) ;
#22495=DIRECTION ( 'NONE',  ( 0.4226182617407188702, 0.000000000000000000, 0.9063077870366409439 ) ) ;
#22497=DIRECTION ( 'NONE',  ( -1.000000000000000000, 0.000000000000000000, 0.000000000000000000 ) ) ;
#22528=ORIENTED_EDGE ( 'NONE', *, *, #5257, .F. ) ;
#22532=ORIENTED_EDGE ( 'NONE', *, *, #12784, .F. ) ;
#22535=FACE_BOUND ( 'NONE', #15118, .T. ) ;
#22550=ORIENTED_EDGE ( 'NONE', *, *, #13548, .F. ) ;
#22559=ORIENTED_EDGE ( 'NONE', *, *, #5201, .T. ) ;
#22572=FACE_OUTER_BOUND ( 'NONE', #23396, .T. ) ;
#22576=FACE_OUTER_BOUND ( 'NONE', #1671, .T. ) ;
#22580=LINE ( 'NONE', #653, #4514 ) ;
#22596=ORIENTED_EDGE ( 'NONE', *, *, #19951, .F. ) ;
#22639=FACE_OUTER_BOUND ( 'NONE', #4814, .T. ) ;
#22695=CARTESIAN_POINT ( 'NONE',  ( -6.637070260807000466, -19.10635214911999924, 2.000000000000000000 ) ) ;
#22704=CARTESIAN_POINT ( 'NONE',  ( -9.000000000000000000, 24.99999999999999645, -6.000000000000000000 ) ) ;
#22710=CARTESIAN_POINT ( 'NONE',  ( -6.095789677045127419, 26.49783382847890678, 1.156958657242621147 ) ) ;
#22715=EDGE_CURVE ( 'NONE', #13647, #15754, #5605, .T. ) ;
#22737=CARTESIAN_POINT ( 'NONE',  ( -9.000000000000000000, 24.99999999999999645, 1.000000000000000000 ) ) ;
#22741=ADVANCED_FACE ( 'NONE', ( #18570 ), #3793, .T. ) ;
#22777=CIRCLE ( 'NONE', #21245, 5.000000000000004441 ) ;
#22815=LINE ( 'NONE', #6105, #5658 ) ;
#22823=ORIENTED_EDGE ( 'NONE', *, *, #13261, .T. ) ;
#22829=CARTESIAN_POINT ( 'NONE',  ( 60.61494135913342518, 35.51856778792605240, 0.000000000000000000 ) ) ;
#22838=ORIENTED_EDGE ( 'NONE', *, *, #4955, .T. ) ;
#22858=CARTESIAN_POINT ( 'NONE',  ( -6.406610618360471854, 27.98165854022565213, 0.9999999999999870104 ) ) ;
#22859=ORIENTED_EDGE ( 'NONE', *, *, #19768, .F. ) ;
#22882=FACE_OUTER_BOUND ( 'NONE', #16046, .T. ) ;
#22883=FACE_OUTER_BOUND ( 'NONE', #16472, .T. ) ;
#22885=ORIENTED_EDGE ( 'NONE', *, *, #7884, .F. ) ;
#22896=VERTEX_POINT ( 'NONE', #860 ) ;
#22897=ORIENTED_EDGE ( 'NONE', *, *, #7317, .F. ) ;
#22989=DIRECTION ( 'NONE',  ( 0.000000000000000000, 1.000000000000000000, 0.000000000000000000 ) ) ;
#22993=ORIENTED_EDGE ( 'NONE', *, *, #17257, .T. ) ;
#23033=EDGE_LOOP ( 'NONE', ( #14142, #6520, #23912, #20759 ) ) ;
#23055=FACE_OUTER_BOUND ( 'NONE', #6694, .T. ) ;
#23121=EDGE_CURVE ( 'NONE', #20808, #7280, #23381, .T. ) ;
#23127=ORIENTED_EDGE ( 'NONE', *, *, #17568, .F. ) ;
#23178=CARTESIAN_POINT ( 'NONE',  ( 44.70988823752291097, 36.26856778792605240, 6.000000000000000000 ) ) ;
#23189=ADVANCED_FACE ( 'NONE', ( #22275 ), #20586, .T. ) ;
#23198=VERTEX_POINT ( 'NONE', #18416 ) ;
#23222=ORIENTED_EDGE ( 'NONE', *, *, #11562, .T. ) ;
#23249=ORIENTED_EDGE ( 'NONE', *, *, #537, .F. ) ;
#23263=CARTESIAN_POINT ( 'NONE',  ( 6.696152422707000618, 26.50000000000000000, -6.000000000000000000 ) ) ;
#23269=PLANE ( 'NONE',  #20689 ) ;
#23276=AXIS2_PLACEMENT_3D ( 'NONE', #15979, #21812, #2929 ) ;
#23281=ORIENTED_EDGE ( 'NONE', *, *, #19133, .F. ) ;
#23320=CARTESIAN_POINT ( 'NONE',  ( -9.000000000000000000, 19.50000000000000000, -2.000000000000000000 ) ) ;
#23345=FACE_OUTER_BOUND ( 'NONE', #1348, .T. ) ;
#23349=LINE ( 'NONE', #408, #7679 ) ;
#23381=LINE ( 'NONE', #1602, #9367 ) ;
#23393=ORIENTED_EDGE ( 'NONE', *, *, #4462, .F. ) ;
#23396=EDGE_LOOP ( 'NONE', ( #4901, #5536, #15105, #205 ) ) ;
#23398=AXIS2_PLACEMENT_3D ( 'NONE', #20011, #3432, #10817 ) ;
#23444=VERTEX_POINT ( 'NONE', #13228 ) ;
#23501=EDGE_CURVE ( 'NONE', #11154, #9971, #11721, .T. ) ;
#23512=ADVANCED_BREP_SHAPE_REPRESENTATION ( '', ( #16570, #4390 ), #11350 ) ;
#23515=DIRECTION ( 'NONE',  ( 0.000000000000000000, 0.000000000000000000, 1.000000000000000000 ) ) ;
#23542=DIRECTION ( 'NONE',  ( -0.5000000000000167644, 0.8660254037844290487, 0.000000000000000000 ) ) ;
#23544=( NAMED_UNIT ( * ) PLANE_ANGLE_UNIT ( ) SI_UNIT ( $, .RADIAN. ) );
#23562=ORIENTED_EDGE ( 'NONE', *, *, #13837, .F. ) ;
#23570=VERTEX_POINT ( 'NONE', #864 ) ;
#23583=CARTESIAN_POINT ( 'NONE',  ( -7.500000000000000000, 24.99999999999999645, -6.000000000000000000 ) ) ;
#23592=AXIS2_PLACEMENT_3D ( 'NONE', #5119, #15751, #4876 ) ;
#23593=EDGE_CURVE ( 'NONE', #17322, #15241, #11781, .T. ) ;
#23616=CARTESIAN_POINT ( 'NONE',  ( 30.87226923053214378, 27.01856778792605240, 2.673746900119611247 ) ) ;
#23624=DIRECTION ( 'NONE',  ( -1.000000000000000000, 0.000000000000000000, 0.000000000000000000 ) ) ;
#23644=DIRECTION ( 'NONE',  ( 0.000000000000000000, 0.000000000000000000, -1.000000000000000000 ) ) ;
#23661=CYLINDRICAL_SURFACE ( 'NONE', #21415, 1.500000000000001332 ) ;
#23685=AXIS2_PLACEMENT_3D ( 'NONE', #141, #7533, #13338 ) ;
#23731=CARTESIAN_POINT ( 'NONE',  ( 21.91677564524291455, 36.61664399927605018, -6.000000000000000000 ) ) ;
#23747=EDGE_CURVE ( 'NONE', #12555, #14083, #4501, .T. ) ;
#23769=EDGE_CURVE ( 'NONE', #23810, #9862, #6192, .T. ) ;
#23776=EDGE_LOOP ( 'NONE', ( #3585, #6770, #11171, #9166, #22182, #10850 ) ) ;
#23778=LINE ( 'NONE', #9250, #10285 ) ;
#23789=VERTEX_POINT ( 'NONE', #4381 ) ;
#23802=APPLICATION_CONTEXT ( 'automotive_design' ) ;
#23810=VERTEX_POINT ( 'NONE', #21706 ) ;
#23826=VECTOR ( 'NONE', #9510, 1000.000000000000000 ) ;
#23834=CARTESIAN_POINT ( 'NONE',  ( -8.250000000000000000, 22.87500000000000000, -6.000000000000000000 ) ) ;
#23856=DIRECTION ( 'NONE',  ( 0.000000000000000000, 0.000000000000000000, 1.000000000000000000 ) ) ;
#23861=CIRCLE ( 'NONE', #13411, 1.500000000000001332 ) ;
#23889=VERTEX_POINT ( 'NONE', #5117 ) ;
#23902=AXIS2_PLACEMENT_3D ( 'NONE', #11873, #19008, #21196 ) ;
#23904=ORIENTED_EDGE ( 'NONE', *, *, #6869, .T. ) ;
#23912=ORIENTED_EDGE ( 'NONE', *, *, #23769, .T. ) ;
#23955=DIRECTION ( 'NONE',  ( 1.000000000000000000, 0.000000000000000000, 0.000000000000000000 ) ) ;
ENDSEC;
END-ISO-10303-21;
